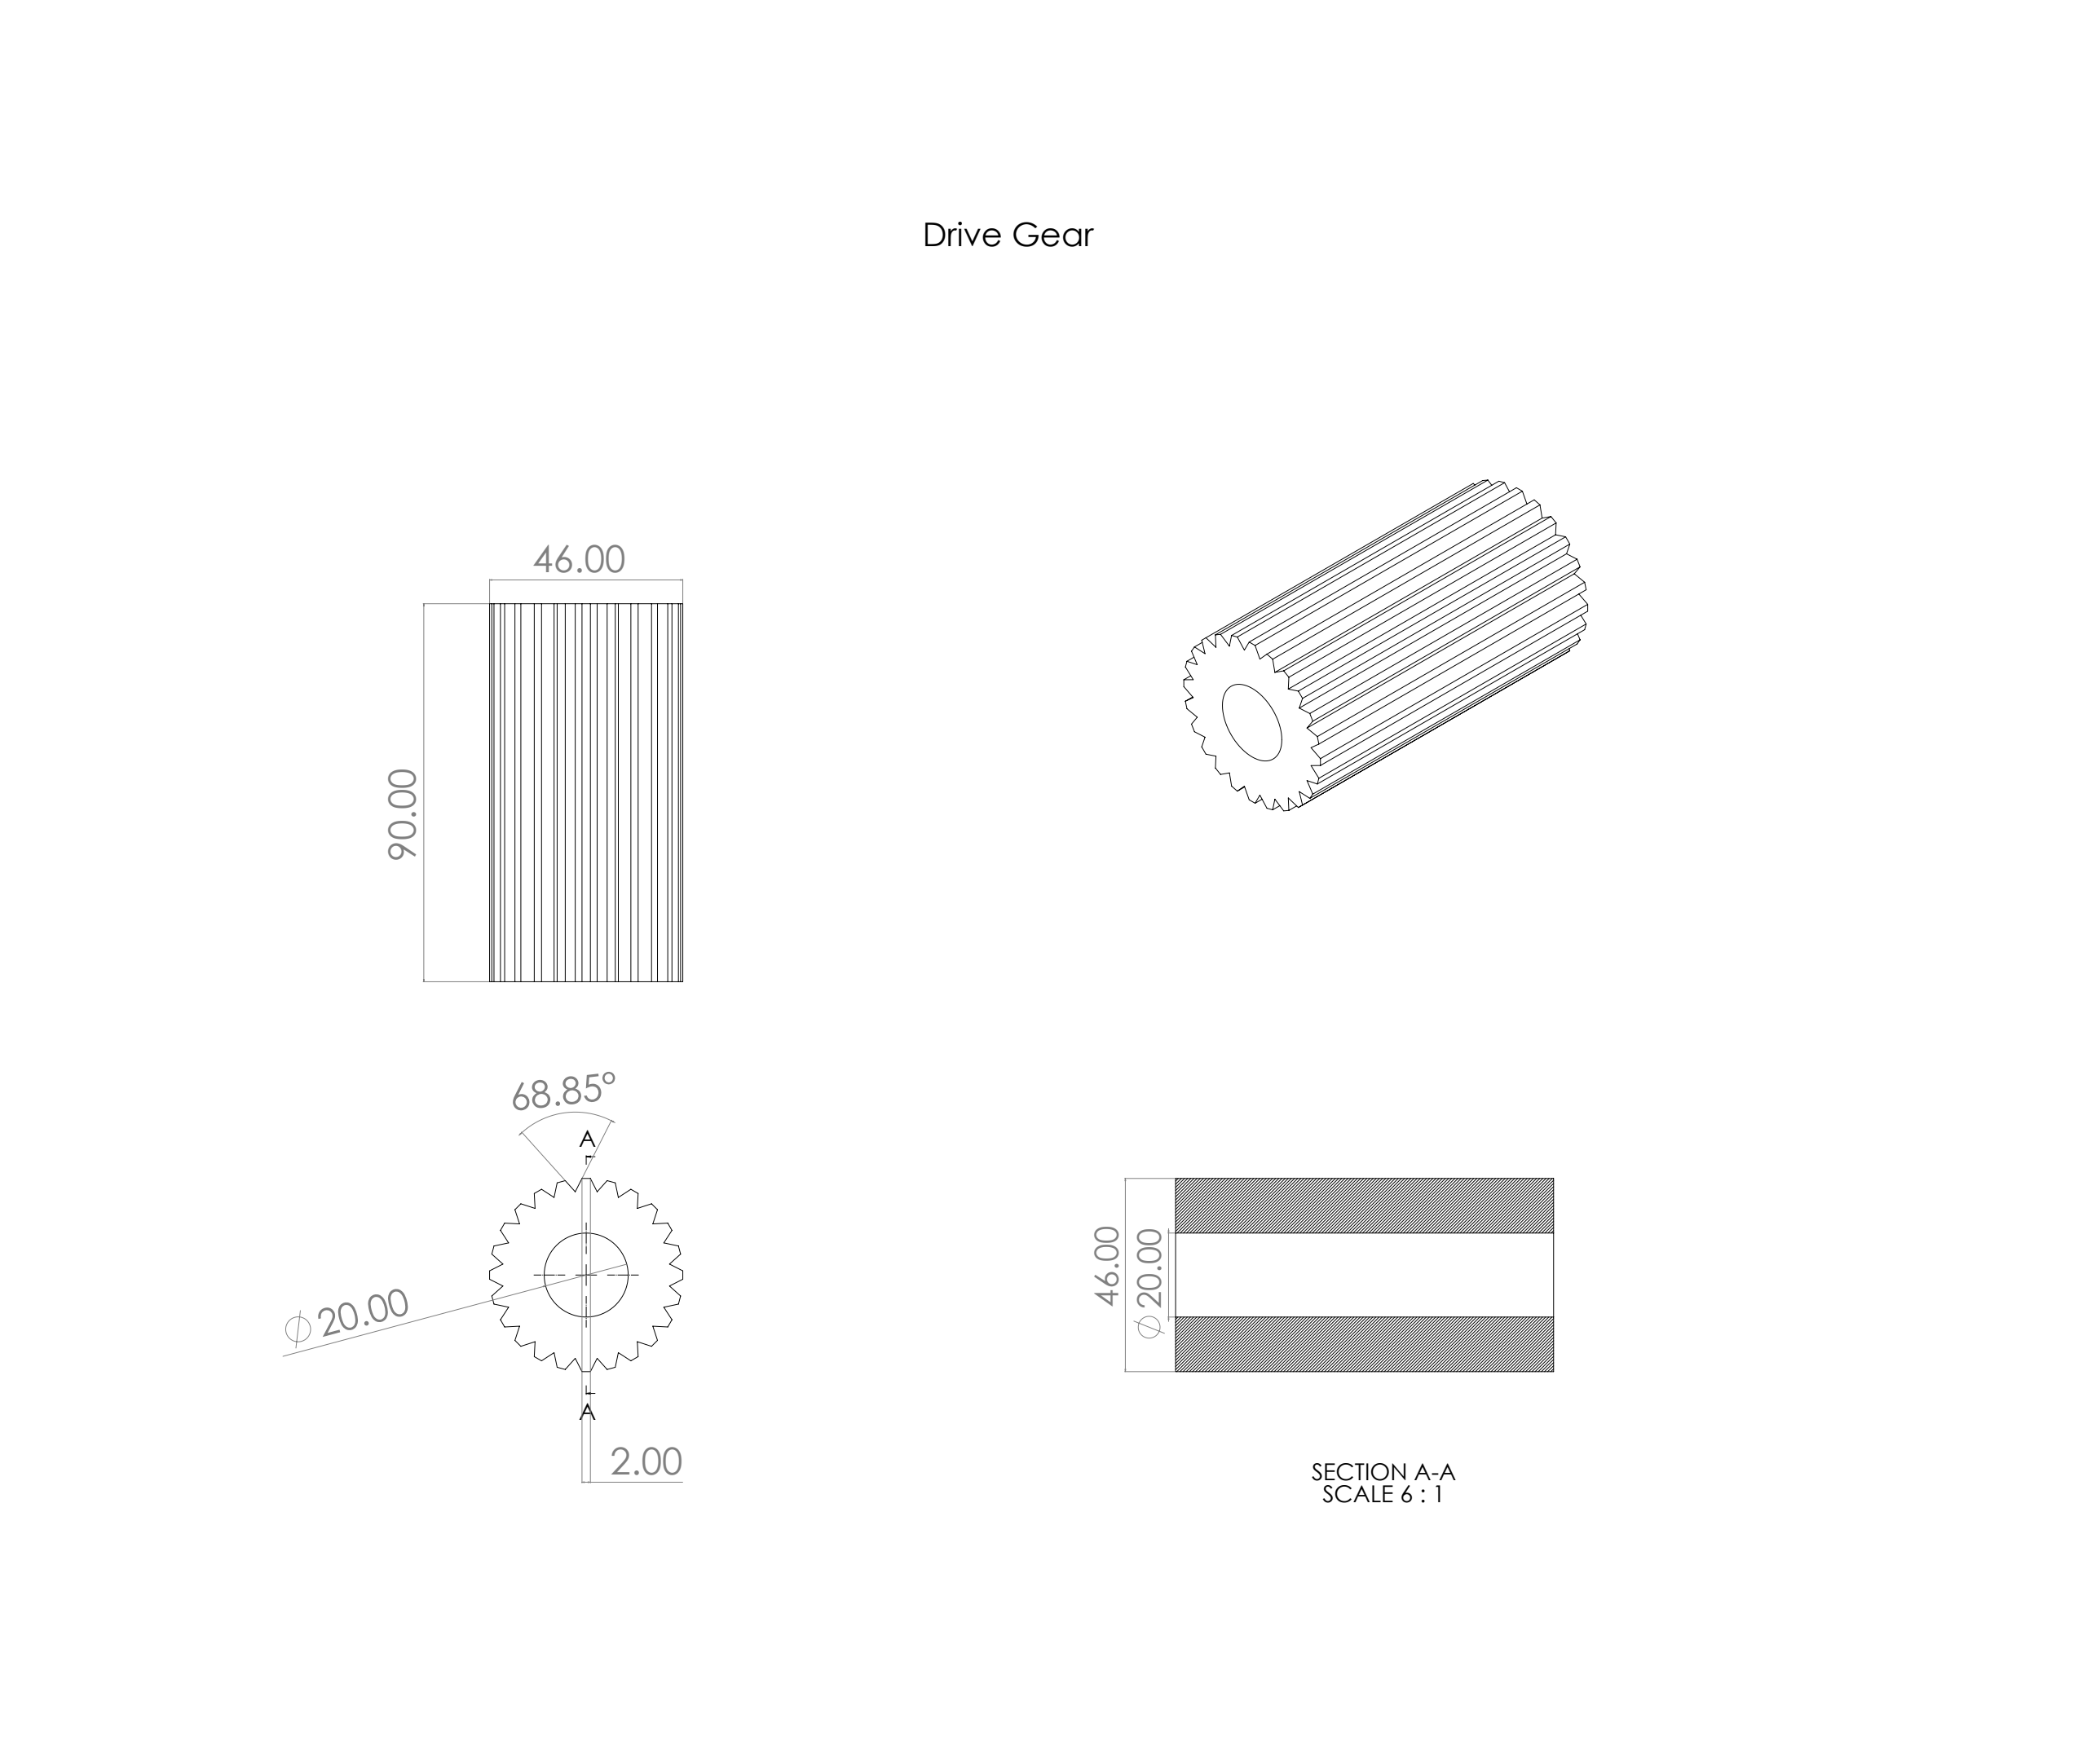
ISO-10303-21;
HEADER;
FILE_DESCRIPTION (('STEP AP214'),
    '1' );
FILE_NAME ('Drive Gear.step',
    '2026-10-24T00:09:50',
    ( '' ),
    ( '' ),
    'SwSTEP 2.0',
    'SolidWorks 2025',
    '' );
FILE_SCHEMA (( 'AUTOMOTIVE_DESIGN' ));
ENDSEC;

DATA;
#40=EDGE_LOOP ( 'NONE', ( #25387, #6950, #12411, #9967 ) ) ;
#42=LINE ( 'NONE', #17847, #25312 ) ;
#78=EDGE_CURVE ( 'NONE', #15009, #7688, #2981, .T. ) ;
#102=LINE ( 'NONE', #19501, #15080 ) ;
#109=EDGE_CURVE ( 'NONE', #28186, #27342, #11484, .T. ) ;
#120=ORIENTED_EDGE ( 'NONE', *, *, #25163, .F. ) ;
#125=PLANE ( 'NONE',  #22915 ) ;
#145=ORIENTED_EDGE ( 'NONE', *, *, #16814, .F. ) ;
#194=VERTEX_POINT ( 'NONE', #10023 ) ;
#196=VECTOR ( 'NONE', #16989, 1000.000000000000000 ) ;
#202=LINE ( 'NONE', #25668, #4520 ) ;
#257=EDGE_LOOP ( 'NONE', ( #18040, #22551, #6751, #26799 ) ) ;
#263=ORIENTED_EDGE ( 'NONE', *, *, #21022, .F. ) ;
#280=CARTESIAN_POINT ( 'NONE',  ( 176.1454027868280434, 57.48855481560072889, -45.00000000000000000 ) ) ;
#290=CARTESIAN_POINT ( 'NONE',  ( 111.3836151241014960, 219.3130464734738325, 45.00000000000000000 ) ) ;
#315=ADVANCED_FACE ( 'NONE', ( #3468 ), #14543, .F. ) ;
#324=CARTESIAN_POINT ( 'NONE',  ( 134.6436608991879496, 206.7391133850113079, 45.00000000000000000 ) ) ;
#338=EDGE_CURVE ( 'NONE', #14636, #5476, #7520, .T. ) ;
#340=EDGE_LOOP ( 'NONE', ( #7547, #3673, #5689, #22912 ) ) ;
#341=ORIENTED_EDGE ( 'NONE', *, *, #16850, .F. ) ;
#343=ADVANCED_FACE ( 'NONE', ( #765 ), #3046, .F. ) ;
#356=AXIS2_PLACEMENT_3D ( 'NONE', #3713, #19096, #27838 ) ;
#395=AXIS2_PLACEMENT_3D ( 'NONE', #17054, #6519, #15304 ) ;
#404=ORIENTED_EDGE ( 'NONE', *, *, #19852, .F. ) ;
#414=VECTOR ( 'NONE', #24913, 999.9999999999998863 ) ;
#421=PLANE ( 'NONE',  #16345 ) ;
#426=CARTESIAN_POINT ( 'NONE',  ( 119.4436508138959567, 203.0294372515225518, 45.00000000000000000 ) ) ;
#460=ORIENTED_EDGE ( 'NONE', *, *, #16342, .F. ) ;
#468=CARTESIAN_POINT ( 'NONE',  ( 157.6866818850739662, 8.471341669691319964, -45.00000000000000000 ) ) ;
#475=DIRECTION ( 'NONE',  ( 0.2066290158914539099, -0.9784193629480814058, 0.000000000000000000 ) ) ;
#481=ORIENTED_EDGE ( 'NONE', *, *, #25209, .F. ) ;
#502=VERTEX_POINT ( 'NONE', #8357 ) ;
#509=ORIENTED_EDGE ( 'NONE', *, *, #9465, .F. ) ;
#551=ORIENTED_EDGE ( 'NONE', *, *, #12670, .T. ) ;
#557=DIRECTION ( 'NONE',  ( -0.9659258262890705327, -0.2588190451025121908, 0.000000000000000000 ) ) ;
#561=CARTESIAN_POINT ( 'NONE',  ( 155.4185842870419947, 230.6339745962152392, -45.00000000000000000 ) ) ;
#570=EDGE_CURVE ( 'NONE', #7917, #3329, #15402, .T. ) ;
#592=AXIS2_PLACEMENT_3D ( 'NONE', #13930, #17784, #13641 ) ;
#599=LINE ( 'NONE', #25008, #4734 ) ;
#609=DIRECTION ( 'NONE',  ( -0.8379557447115514313, 0.5457381880580733924, 0.000000000000000000 ) ) ;
#612=ORIENTED_EDGE ( 'NONE', *, *, #27121, .T. ) ;
#617=LINE ( 'NONE', #13264, #2052 ) ;
#626=CARTESIAN_POINT ( 'NONE',  ( 0.000000000000000000, 0.000000000000000000, 45.00000000000000000 ) ) ;
#627=VERTEX_POINT ( 'NONE', #26725 ) ;
#641=ORIENTED_EDGE ( 'NONE', *, *, #2045, .T. ) ;
#642=LINE ( 'NONE', #11850, #26984 ) ;
#649=LINE ( 'NONE', #27065, #16667 ) ;
#686=CARTESIAN_POINT ( 'NONE',  ( 122.8247714198253959, 235.8670668058242939, 45.00000000000000000 ) ) ;
#694=ORIENTED_EDGE ( 'NONE', *, *, #13779, .T. ) ;
#706=CARTESIAN_POINT ( 'NONE',  ( -56.65306767071049165, 63.08575069354419185, 45.00000000000000000 ) ) ;
#716=AXIS2_PLACEMENT_3D ( 'NONE', #20523, #18375, #3692 ) ;
#718=DIRECTION ( 'NONE',  ( 0.9985600561963489108, -0.05364526231778980747, 0.000000000000000000 ) ) ;
#720=PLANE ( 'NONE',  #20781 ) ;
#732=VECTOR ( 'NONE', #22180, 1000.000000000000000 ) ;
#740=CARTESIAN_POINT ( 'NONE',  ( 145.6339745962154097, 240.4185842870418242, 45.00000000000000000 ) ) ;
#765=FACE_OUTER_BOUND ( 'NONE', #3853, .T. ) ;
#781=DIRECTION ( 'NONE',  ( 0.7071067811865474617, 0.7071067811865474617, 0.000000000000000000 ) ) ;
#788=PLANE ( 'NONE',  #25217 ) ;
#803=ORIENTED_EDGE ( 'NONE', *, *, #16888, .F. ) ;
#809=LINE ( 'NONE', #11602, #22008 ) ;
#810=VECTOR ( 'NONE', #4848, 1000.000000000000000 ) ;
#825=VECTOR ( 'NONE', #26696, 1000.000000000000000 ) ;
#860=VERTEX_POINT ( 'NONE', #14376 ) ;
#884=CARTESIAN_POINT ( 'NONE',  ( -26.22291647523108438, 23.54903675176048594, -45.00000000000000000 ) ) ;
#894=EDGE_CURVE ( 'NONE', #10441, #6349, #7345, .T. ) ;
#900=EDGE_CURVE ( 'NONE', #19228, #8289, #8468, .T. ) ;
#916=VECTOR ( 'NONE', #2379, 1000.000000000000114 ) ;
#950=FACE_OUTER_BOUND ( 'NONE', #5628, .T. ) ;
#951=FACE_OUTER_BOUND ( 'NONE', #17284, .T. ) ;
#953=LINE ( 'NONE', #18483, #6794 ) ;
#962=VERTEX_POINT ( 'NONE', #1425 ) ;
#963=VECTOR ( 'NONE', #22515, 1000.000000000000000 ) ;
#994=CARTESIAN_POINT ( 'NONE',  ( -55.40193461144291831, 169.7519813918499665, 45.00000000000000000 ) ) ;
#999=VERTEX_POINT ( 'NONE', #1707 ) ;
#1002=DIRECTION ( 'NONE',  ( -0.000000000000000000, -0.000000000000000000, -1.000000000000000000 ) ) ;
#1028=ORIENTED_EDGE ( 'NONE', *, *, #14203, .T. ) ;
#1040=ORIENTED_EDGE ( 'NONE', *, *, #11015, .F. ) ;
#1048=CARTESIAN_POINT ( 'NONE',  ( 116.5224093497741364, 227.6536686473013447, 45.00000000000000000 ) ) ;
#1079=EDGE_LOOP ( 'NONE', ( #25472, #803, #15589, #7233 ) ) ;
#1083=ADVANCED_FACE ( 'NONE', ( #13352 ), #125, .F. ) ;
#1084=CARTESIAN_POINT ( 'NONE',  ( 111.9999999999999289, 218.9999999999996874, 45.00000000000000000 ) ) ;
#1090=DIRECTION ( 'NONE',  ( -0.9784193629480828491, -0.2066290158914464437, 0.000000000000000000 ) ) ;
#1092=CARTESIAN_POINT ( 'NONE',  ( -56.65306767071049165, 63.08575069354419185, -45.00000000000000000 ) ) ;
#1094=VECTOR ( 'NONE', #24258, 1000.000000000000000 ) ;
#1102=ORIENTED_EDGE ( 'NONE', *, *, #26834, .F. ) ;
#1115=CARTESIAN_POINT ( 'NONE',  ( -15.28840184913744515, 9.956927649352207865, -45.00000000000000000 ) ) ;
#1118=VECTOR ( 'NONE', #26590, 1000.000000000000114 ) ;
#1121=DIRECTION ( 'NONE',  ( 0.8379557447115634217, 0.5457381880580551847, -0.000000000000000000 ) ) ;
#1126=DIRECTION ( 'NONE',  ( -0.9659258262890652036, 0.2588190451025321748, 0.000000000000000000 ) ) ;
#1135=LINE ( 'NONE', #994, #11133 ) ;
#1148=VECTOR ( 'NONE', #9574, 1000.000000000000000 ) ;
#1152=LINE ( 'NONE', #23410, #5980 ) ;
#1163=DIRECTION ( 'NONE',  ( 0.05364526231778980747, 0.9985600561963489108, -0.000000000000000000 ) ) ;
#1183=DIRECTION ( 'NONE',  ( 0.9506505318133497973, -0.3102637045530707294, 0.000000000000000000 ) ) ;
#1209=ORIENTED_EDGE ( 'NONE', *, *, #3052, .T. ) ;
#1216=EDGE_CURVE ( 'NONE', #7652, #26924, #15939, .T. ) ;
#1218=ORIENTED_EDGE ( 'NONE', *, *, #16788, .T. ) ;
#1234=VECTOR ( 'NONE', #20751, 1000.000000000000000 ) ;
#1238=CARTESIAN_POINT ( 'NONE',  ( 133.9999999999998295, 242.9999999999997158, 45.00000000000000000 ) ) ;
#1259=CARTESIAN_POINT ( 'NONE',  ( 81.39309752945497678, 249.3891174404998594, -45.00000000000000000 ) ) ;
#1260=FACE_OUTER_BOUND ( 'NONE', #1079, .T. ) ;
#1267=ORIENTED_EDGE ( 'NONE', *, *, #22908, .T. ) ;
#1274=CIRCLE ( 'NONE', #5845, 10.00000000000000888 ) ;
#1279=EDGE_LOOP ( 'NONE', ( #24711, #16218, #9881, #10613 ) ) ;
#1302=LINE ( 'NONE', #3588, #3177 ) ;
#1318=DIRECTION ( 'NONE',  ( -0.4999999999999865108, 0.8660254037844464792, 0.000000000000000000 ) ) ;
#1339=EDGE_CURVE ( 'NONE', #6712, #11692, #8855, .T. ) ;
#1341=ADVANCED_FACE ( 'NONE', ( #10873 ), #11018, .F. ) ;
#1345=CARTESIAN_POINT ( 'NONE',  ( 130.0130877889311591, 197.5248869502486571, 45.00000000000000000 ) ) ;
#1355=ORIENTED_EDGE ( 'NONE', *, *, #570, .F. ) ;
#1361=EDGE_LOOP ( 'NONE', ( #16416, #481, #3606, #1446 ) ) ;
#1388=CARTESIAN_POINT ( 'NONE',  ( -54.22951502486254327, 83.26691194124390449, -45.00000000000000000 ) ) ;
#1389=ORIENTED_EDGE ( 'NONE', *, *, #3470, .F. ) ;
#1416=EDGE_LOOP ( 'NONE', ( #15996, #14532, #28328, #12988 ) ) ;
#1418=EDGE_LOOP ( 'NONE', ( #12140, #21492, #17241, #7648 ) ) ;
#1421=ORIENTED_EDGE ( 'NONE', *, *, #8652, .T. ) ;
#1425=CARTESIAN_POINT ( 'NONE',  ( 127.3463313526982716, 201.5224093497739943, 45.00000000000000000 ) ) ;
#1426=DIRECTION ( 'NONE',  ( -0.8660254037844454800, -0.4999999999999881206, 0.000000000000000000 ) ) ;
#1427=DIRECTION ( 'NONE',  ( -0.000000000000000000, -0.000000000000000000, -1.000000000000000000 ) ) ;
#1446=ORIENTED_EDGE ( 'NONE', *, *, #16888, .T. ) ;
#1449=LINE ( 'NONE', #22871, #12208 ) ;
#1466=EDGE_CURVE ( 'NONE', #27470, #21163, #18610, .T. ) ;
#1478=VECTOR ( 'NONE', #2911, 1000.000000000000114 ) ;
#1485=ORIENTED_EDGE ( 'NONE', *, *, #25059, .F. ) ;
#1487=LINE ( 'NONE', #27761, #26260 ) ;
#1498=ORIENTED_EDGE ( 'NONE', *, *, #13064, .T. ) ;
#1530=ORIENTED_EDGE ( 'NONE', *, *, #23337, .F. ) ;
#1551=DIRECTION ( 'NONE',  ( 0.2066290158914464714, -0.9784193629480829602, 0.000000000000000000 ) ) ;
#1553=DIRECTION ( 'NONE',  ( -0.000000000000000000, -0.000000000000000000, -1.000000000000000000 ) ) ;
#1554=VERTEX_POINT ( 'NONE', #1084 ) ;
#1596=ORIENTED_EDGE ( 'NONE', *, *, #15234, .T. ) ;
#1606=PLANE ( 'NONE',  #14436 ) ;
#1621=CARTESIAN_POINT ( 'NONE',  ( 147.1752285801744904, 204.1329331941753082, -45.00000000000000000 ) ) ;
#1629=DIRECTION ( 'NONE',  ( -0.000000000000000000, -0.000000000000000000, -1.000000000000000000 ) ) ;
#1631=ORIENTED_EDGE ( 'NONE', *, *, #5242, .F. ) ;
#1636=ORIENTED_EDGE ( 'NONE', *, *, #26899, .F. ) ;
#1650=CARTESIAN_POINT ( 'NONE',  ( 177.1897033089359184, 197.3087408678716770, 45.00000000000000000 ) ) ;
#1666=DIRECTION ( 'NONE',  ( -0.9784193629480785193, 0.2066290158914672603, 0.000000000000000000 ) ) ;
#1704=ORIENTED_EDGE ( 'NONE', *, *, #7266, .T. ) ;
#1707=CARTESIAN_POINT ( 'NONE',  ( 144.9999999999998863, 220.0000000000000284, -45.00000000000000000 ) ) ;
#1719=ORIENTED_EDGE ( 'NONE', *, *, #1339, .T. ) ;
#1736=VERTEX_POINT ( 'NONE', #1916 ) ;
#1748=CIRCLE ( 'NONE', #20114, 10.00000000000000888 ) ;
#1754=EDGE_CURVE ( 'NONE', #18948, #27470, #15575, .T. ) ;
#1758=SHAPE_REPRESENTATION_RELATIONSHIP ( 'NONE' , 'NONE' ,  #18912, #11228 ) ;
#1763=VECTOR ( 'NONE', #14890, 1000.000000000000000 ) ;
#1765=EDGE_LOOP ( 'NONE', ( #4521, #6128, #4628, #3710 ) ) ;
#1782=VECTOR ( 'NONE', #5929, 1000.000000000000000 ) ;
#1791=LINE ( 'NONE', #13023, #4249 ) ;
#1844=ADVANCED_FACE ( 'NONE', ( #4356 ), #17291, .F. ) ;
#1868=LINE ( 'NONE', #10646, #5333 ) ;
#1869=ORIENTED_EDGE ( 'NONE', *, *, #5831, .T. ) ;
#1870=ORIENTED_EDGE ( 'NONE', *, *, #3281, .F. ) ;
#1885=AXIS2_PLACEMENT_3D ( 'NONE', #20179, #11860, #26790 ) ;
#1887=VECTOR ( 'NONE', #26855, 1000.000000000000114 ) ;
#1892=DIRECTION ( 'NONE',  ( 0.5457381880580697286, -0.8379557447115539848, 0.000000000000000000 ) ) ;
#1897=DIRECTION ( 'NONE',  ( 1.000000000000000000, 0.000000000000000000, 0.000000000000000000 ) ) ;
#1916=CARTESIAN_POINT ( 'NONE',  ( 119.1329331941753225, 207.8247714198252254, -45.00000000000000000 ) ) ;
#1918=CARTESIAN_POINT ( 'NONE',  ( 67.86343429515802939, -22.14858123305036486, -45.00000000000000000 ) ) ;
#1945=EDGE_LOOP ( 'NONE', ( #6961, #13309, #1870, #11630 ) ) ;
#1974=EDGE_LOOP ( 'NONE', ( #18192, #8711 ) ) ;
#1976=AXIS2_PLACEMENT_3D ( 'NONE', #3956, #4099, #27934 ) ;
#2037=PLANE ( 'NONE',  #3279 ) ;
#2045=EDGE_CURVE ( 'NONE', #27342, #12331, #5777, .T. ) ;
#2052=VECTOR ( 'NONE', #18137, 1000.000000000000114 ) ;
#2068=LINE ( 'NONE', #20020, #17266 ) ;
#2075=ADVANCED_FACE ( 'NONE', ( #9953 ), #7662, .F. ) ;
#2089=ORIENTED_EDGE ( 'NONE', *, *, #3406, .F. ) ;
#2117=APPLICATION_CONTEXT ( 'automotive_design' ) ;
#2121=DIRECTION ( 'NONE',  ( -0.9659258262890705327, -0.2588190451025121908, 0.000000000000000000 ) ) ;
#2154=EDGE_CURVE ( 'NONE', #11738, #18634, #27740, .T. ) ;
#2166=ADVANCED_FACE ( 'NONE', ( #14689 ), #9817, .F. ) ;
#2189=ORIENTED_EDGE ( 'NONE', *, *, #1216, .T. ) ;
#2192=VECTOR ( 'NONE', #13945, 1000.000000000000114 ) ;
#2198=DIRECTION ( 'NONE',  ( 1.000000000000000000, 0.000000000000000000, 0.000000000000000000 ) ) ;
#2203=DIRECTION ( 'NONE',  ( 0.9985600561963492439, 0.05364526231778202897, 0.000000000000000000 ) ) ;
#2230=VECTOR ( 'NONE', #25058, 1000.000000000000000 ) ;
#2232=ADVANCED_FACE ( 'NONE', ( #15658 ), #421, .F. ) ;
#2234=EDGE_CURVE ( 'NONE', #24120, #14926, #7170, .T. ) ;
#2235=CARTESIAN_POINT ( 'NONE',  ( 111.3836151241014960, 219.3130464734738325, -45.00000000000000000 ) ) ;
#2237=PLANE ( 'NONE',  #21348 ) ;
#2246=ORIENTED_EDGE ( 'NONE', *, *, #12352, .F. ) ;
#2288=ORIENTED_EDGE ( 'NONE', *, *, #3470, .T. ) ;
#2320=DIRECTION ( 'NONE',  ( 0.000000000000000000, 0.000000000000000000, 1.000000000000000000 ) ) ;
#2324=CARTESIAN_POINT ( 'NONE',  ( 69.99612328191057031, 261.2290884209365345, -45.00000000000000000 ) ) ;
#2379=DIRECTION ( 'NONE',  ( 0.8916010070293484135, -0.4528218681382910060, 0.000000000000000000 ) ) ;
#2401=EDGE_CURVE ( 'NONE', #25350, #8917, #22540, .T. ) ;
#2412=DIRECTION ( 'NONE',  ( 0.6681556583950086781, -0.7440215159219069063, 0.000000000000000000 ) ) ;
#2417=VECTOR ( 'NONE', #27846, 1000.000000000000000 ) ;
#2447=DIRECTION ( 'NONE',  ( -0.9985600561963481336, 0.05364526231780537141, 0.000000000000000000 ) ) ;
#2471=CARTESIAN_POINT ( 'NONE',  ( 8.415662294793918363, -4.274104551145060604, 45.00000000000000000 ) ) ;
#2476=VECTOR ( 'NONE', #18133, 1000.000000000000000 ) ;
#2490=ORIENTED_EDGE ( 'NONE', *, *, #5540, .T. ) ;
#2507=ADVANCED_FACE ( 'NONE', ( #21795 ), #2237, .F. ) ;
#2519=LINE ( 'NONE', #2235, #916 ) ;
#2554=UNCERTAINTY_MEASURE_WITH_UNIT (LENGTH_MEASURE( 1.000000000000000082E-05 ), #11582, 'distance_accuracy_value', 'NONE');
#2558=DIRECTION ( 'NONE',  ( 0.3102637045530588500, -0.9506505318133536830, 0.000000000000000000 ) ) ;
#2564=LINE ( 'NONE', #426, #825 ) ;
#2570=DIRECTION ( 'NONE',  ( -0.000000000000000000, -0.000000000000000000, -1.000000000000000000 ) ) ;
#2571=DIRECTION ( 'NONE',  ( -0.8660254037844394848, 0.4999999999999985012, 0.000000000000000000 ) ) ;
#2580=AXIS2_PLACEMENT_3D ( 'NONE', #15107, #13103, #3886 ) ;
#2587=ORIENTED_EDGE ( 'NONE', *, *, #26111, .F. ) ;
#2592=CARTESIAN_POINT ( 'NONE',  ( 161.2365440327092472, 161.2365440327092472, 45.00000000000000000 ) ) ;
#2611=VERTEX_POINT ( 'NONE', #23070 ) ;
#2612=CARTESIAN_POINT ( 'NONE',  ( 119.4436508138959567, 203.0294372515225518, -45.00000000000000000 ) ) ;
#2654=ORIENTED_EDGE ( 'NONE', *, *, #23931, .T. ) ;
#2666=DIRECTION ( 'NONE',  ( 0.2066290158914672881, 0.9784193629480785193, 0.000000000000000000 ) ) ;
#2679=EDGE_CURVE ( 'NONE', #24350, #28016, #12165, .T. ) ;
#2681=LINE ( 'NONE', #5123, #20173 ) ;
#2710=CARTESIAN_POINT ( 'NONE',  ( 122.8247714198256944, 204.1329331941749672, 45.00000000000000000 ) ) ;
#2712=VECTOR ( 'NONE', #22898, 999.9999999999998863 ) ;
#2721=VECTOR ( 'NONE', #7878, 1000.000000000000000 ) ;
#2725=VECTOR ( 'NONE', #21249, 999.9999999999998863 ) ;
#2732=ADVANCED_FACE ( 'NONE', ( #20765 ), #9855, .F. ) ;
#2745=LINE ( 'NONE', #18132, #9284 ) ;
#2746=LINE ( 'NONE', #7067, #18086 ) ;
#2762=DIRECTION ( 'NONE',  ( 0.9985600561963485777, -0.05364526231779676024, 0.000000000000000000 ) ) ;
#2779=CARTESIAN_POINT ( 'NONE',  ( 132.3894761555990556, 200.1711027725235397, 45.00000000000000000 ) ) ;
#2780=DIRECTION ( 'NONE',  ( -0.7071067811865614505, -0.7071067811865336949, 0.000000000000000000 ) ) ;
#2792=ORIENTED_EDGE ( 'NONE', *, *, #22790, .F. ) ;
#2801=CARTESIAN_POINT ( 'NONE',  ( 157.9999999999998579, 219.0000000000000284, -45.00000000000000000 ) ) ;
#2814=DIRECTION ( 'NONE',  ( -0.9659258262890670910, 0.2588190451025251804, 0.000000000000000000 ) ) ;
#2817=PLANE ( 'NONE',  #28111 ) ;
#2823=LINE ( 'NONE', #11617, #23613 ) ;
#2845=LINE ( 'NONE', #20656, #9838 ) ;
#2847=LINE ( 'NONE', #11639, #4974 ) ;
#2850=CARTESIAN_POINT ( 'NONE',  ( 151.9705627484769650, 235.5563491861038017, 45.00000000000000000 ) ) ;
#2870=ORIENTED_EDGE ( 'NONE', *, *, #14550, .T. ) ;
#2873=VERTEX_POINT ( 'NONE', #10139 ) ;
#2890=EDGE_CURVE ( 'NONE', #24769, #999, #18891, .T. ) ;
#2902=FACE_OUTER_BOUND ( 'NONE', #28230, .T. ) ;
#2910=ORIENTED_EDGE ( 'NONE', *, *, #25628, .T. ) ;
#2911=DIRECTION ( 'NONE',  ( 0.05364526231776645809, -0.9985600561963501320, 0.000000000000000000 ) ) ;
#2925=DIRECTION ( 'NONE',  ( -0.000000000000000000, -0.000000000000000000, -1.000000000000000000 ) ) ;
#2927=CARTESIAN_POINT ( 'NONE',  ( 46.36636626309694975, -15.13258561588589757, -45.00000000000000000 ) ) ;
#2930=DIRECTION ( 'NONE',  ( 0.2588190451024993122, -0.9659258262890740854, 0.000000000000000000 ) ) ;
#2939=VERTEX_POINT ( 'NONE', #15446 ) ;
#2940=DIRECTION ( 'NONE',  ( -0.000000000000000000, -0.000000000000000000, -1.000000000000000000 ) ) ;
#2968=DIRECTION ( 'NONE',  ( -0.000000000000000000, -0.000000000000000000, -1.000000000000000000 ) ) ;
#2976=ORIENTED_EDGE ( 'NONE', *, *, #25059, .T. ) ;
#2981=LINE ( 'NONE', #7160, #15959 ) ;
#2988=DIRECTION ( 'NONE',  ( -0.000000000000000000, -0.000000000000000000, -1.000000000000000000 ) ) ;
#3005=EDGE_CURVE ( 'NONE', #27691, #16717, #15580, .T. ) ;
#3015=VECTOR ( 'NONE', #6084, 1000.000000000000000 ) ;
#3035=ORIENTED_EDGE ( 'NONE', *, *, #2045, .F. ) ;
#3046=PLANE ( 'NONE',  #15104 ) ;
#3052=EDGE_CURVE ( 'NONE', #24120, #16717, #26777, .T. ) ;
#3063=DIRECTION ( 'NONE',  ( -0.4999999999999985012, -0.8660254037844394848, 0.000000000000000000 ) ) ;
#3070=ORIENTED_EDGE ( 'NONE', *, *, #1754, .F. ) ;
#3088=CIRCLE ( 'NONE', #356, 10.00000000000000888 ) ;
#3091=CARTESIAN_POINT ( 'NONE',  ( 193.7634559672933676, 193.7634559672857790, 45.00000000000000000 ) ) ;
#3092=CARTESIAN_POINT ( 'NONE',  ( -26.23654403271235225, 26.23654403271337543, 45.00000000000000000 ) ) ;
#3123=VECTOR ( 'NONE', #22798, 1000.000000000000000 ) ;
#3133=DIRECTION ( 'NONE',  ( 0.000000000000000000, -0.000000000000000000, -1.000000000000000000 ) ) ;
#3138=DIRECTION ( 'NONE',  ( -0.9985600561963485777, -0.05364526231779759985, 0.000000000000000000 ) ) ;
#3157=VECTOR ( 'NONE', #2121, 1000.000000000000114 ) ;
#3177=VECTOR ( 'NONE', #21120, 1000.000000000000114 ) ;
#3182=FACE_OUTER_BOUND ( 'NONE', #20955, .T. ) ;
#3242=LINE ( 'NONE', #18765, #15841 ) ;
#3264=CARTESIAN_POINT ( 'NONE',  ( 185.9255560592262100, 121.0883471088020116, 45.00000000000000000 ) ) ;
#3279=AXIS2_PLACEMENT_3D ( 'NONE', #8516, #21866, #17268 ) ;
#3281=EDGE_CURVE ( 'NONE', #10285, #27697, #26871, .T. ) ;
#3300=EDGE_CURVE ( 'NONE', #7395, #1554, #9777, .T. ) ;
#3309=EDGE_CURVE ( 'NONE', #7097, #3365, #25132, .T. ) ;
#3311=PLANE ( 'NONE',  #21814 ) ;
#3326=DIRECTION ( 'NONE',  ( 1.387778780781444413E-14, 1.000000000000000000, 0.000000000000000000 ) ) ;
#3329=VERTEX_POINT ( 'NONE', #17790 ) ;
#3334=CARTESIAN_POINT ( 'NONE',  ( -43.04748092857122543, 38.65804596583237895, 45.00000000000000000 ) ) ;
#3339=EDGE_CURVE ( 'NONE', #20334, #27997, #18371, .T. ) ;
#3342=DIRECTION ( 'NONE',  ( -0.7440215159219069063, -0.6681556583950086781, 0.000000000000000000 ) ) ;
#3343=LINE ( 'NONE', #10247, #5075 ) ;
#3350=VERTEX_POINT ( 'NONE', #24402 ) ;
#3365=VERTEX_POINT ( 'NONE', #22247 ) ;
#3369=VECTOR ( 'NONE', #15588, 1000.000000000000000 ) ;
#3376=ADVANCED_FACE ( 'NONE', ( #22106 ), #6876, .F. ) ;
#3405=VECTOR ( 'NONE', #9865, 1000.000000000000000 ) ;
#3406=EDGE_CURVE ( 'NONE', #26858, #28003, #5000, .T. ) ;
#3410=CARTESIAN_POINT ( 'NONE',  ( 119.4436508138957720, 236.9705627484767376, 45.00000000000000000 ) ) ;
#3415=FACE_OUTER_BOUND ( 'NONE', #6007, .T. ) ;
#3421=ORIENTED_EDGE ( 'NONE', *, *, #26111, .T. ) ;
#3439=EDGE_CURVE ( 'NONE', #1554, #13479, #2847, .T. ) ;
#3460=EDGE_CURVE ( 'NONE', #16717, #18830, #27813, .T. ) ;
#3468=FACE_OUTER_BOUND ( 'NONE', #28210, .T. ) ;
#3470=EDGE_CURVE ( 'NONE', #21880, #27997, #25394, .T. ) ;
#3472=ORIENTED_EDGE ( 'NONE', *, *, #26710, .T. ) ;
#3475=EDGE_CURVE ( 'NONE', #3728, #10441, #23379, .T. ) ;
#3496=VERTEX_POINT ( 'NONE', #9889 ) ;
#3512=ADVANCED_FACE ( 'NONE', ( #1260 ), #16502, .F. ) ;
#3523=EDGE_LOOP ( 'NONE', ( #17931, #11794, #13410, #15572 ) ) ;
#3524=DIRECTION ( 'NONE',  ( 0.9985600561963481336, -0.05364526231780537141, 0.000000000000000000 ) ) ;
#3531=PLANE ( 'NONE',  #11762 ) ;
#3554=CARTESIAN_POINT ( 'NONE',  ( -26.23654403271235225, 26.23654403271337543, -45.00000000000000000 ) ) ;
#3561=VECTOR ( 'NONE', #21819, 1000.000000000000000 ) ;
#3579=DIRECTION ( 'NONE',  ( -0.000000000000000000, -0.000000000000000000, -1.000000000000000000 ) ) ;
#3585=CARTESIAN_POINT ( 'NONE',  ( 150.8670668058245212, 232.1752285801742630, 45.00000000000000000 ) ) ;
#3588=CARTESIAN_POINT ( 'NONE',  ( -43.04748092857122543, 38.65804596583237895, -45.00000000000000000 ) ) ;
#3606=ORIENTED_EDGE ( 'NONE', *, *, #18957, .F. ) ;
#3613=CARTESIAN_POINT ( 'NONE',  ( 115.1711027725237955, 217.3894761555985156, -45.00000000000000000 ) ) ;
#3639=EDGE_CURVE ( 'NONE', #22969, #27280, #17578, .T. ) ;
#3640=VECTOR ( 'NONE', #17767, 1000.000000000000114 ) ;
#3649=VERTEX_POINT ( 'NONE', #13151 ) ;
#3666=EDGE_CURVE ( 'NONE', #15219, #4484, #202, .T. ) ;
#3673=ORIENTED_EDGE ( 'NONE', *, *, #23039, .F. ) ;
#3674=EDGE_CURVE ( 'NONE', #24234, #24769, #1748, .T. ) ;
#3677=ORIENTED_EDGE ( 'NONE', *, *, #15337, .F. ) ;
#3682=ORIENTED_EDGE ( 'NONE', *, *, #11254, .T. ) ;
#3687=DIRECTION ( 'NONE',  ( -0.000000000000000000, -0.000000000000000000, -1.000000000000000000 ) ) ;
#3692=DIRECTION ( 'NONE',  ( 0.8916010070293515222, -0.4528218681382848443, 0.000000000000000000 ) ) ;
#3710=ORIENTED_EDGE ( 'NONE', *, *, #8134, .T. ) ;
#3713=CARTESIAN_POINT ( 'NONE',  ( 134.9999999999998579, 220.0000000000000284, 45.00000000000000000 ) ) ;
#3717=EDGE_CURVE ( 'NONE', #6540, #10285, #26468, .T. ) ;
#3728=VERTEX_POINT ( 'NONE', #22322 ) ;
#3744=AXIS2_PLACEMENT_3D ( 'NONE', #15881, #2780, #28028 ) ;
#3756=FACE_OUTER_BOUND ( 'NONE', #11512, .T. ) ;
#3759=ADVANCED_FACE ( 'NONE', ( #10449 ), #19207, .F. ) ;
#3786=ORIENTED_EDGE ( 'NONE', *, *, #2679, .F. ) ;
#3811=CARTESIAN_POINT ( 'NONE',  ( 0.000000000000000000, 196.9999999999997442, 45.00000000000000000 ) ) ;
#3843=PLANE ( 'NONE',  #16875 ) ;
#3848=CARTESIAN_POINT ( 'NONE',  ( 157.4751130497510303, 215.0130877889310455, -45.00000000000000000 ) ) ;
#3850=ORIENTED_EDGE ( 'NONE', *, *, #17554, .T. ) ;
#3853=EDGE_LOOP ( 'NONE', ( #11519, #4209, #23044, #8212 ) ) ;
#3880=VERTEX_POINT ( 'NONE', #13717 ) ;
#3885=CARTESIAN_POINT ( 'NONE',  ( 113.0425250404539241, 213.0812361363525440, -45.00000000000000000 ) ) ;
#3886=DIRECTION ( 'NONE',  ( 0.000000000000000000, 0.000000000000000000, 1.000000000000000000 ) ) ;
#3899=CARTESIAN_POINT ( 'NONE',  ( 12.78000883847031588, 237.8887863075477469, 45.00000000000000000 ) ) ;
#3915=DIRECTION ( 'NONE',  ( -0.000000000000000000, -0.000000000000000000, -1.000000000000000000 ) ) ;
#3917=ORIENTED_EDGE ( 'NONE', *, *, #27423, .F. ) ;
#3928=DIRECTION ( 'NONE',  ( -0.8660254037844326014, 0.5000000000000106581, 0.000000000000000000 ) ) ;
#3947=ORIENTED_EDGE ( 'NONE', *, *, #18957, .T. ) ;
#3949=FACE_OUTER_BOUND ( 'NONE', #13104, .T. ) ;
#3953=CARTESIAN_POINT ( 'NONE',  ( 58.09044720719344213, 216.7965004116395562, -45.00000000000000000 ) ) ;
#3956=CARTESIAN_POINT ( 'NONE',  ( -50.01279441628821587, 86.62470095750859400, 45.00000000000000000 ) ) ;
#3965=ORIENTED_EDGE ( 'NONE', *, *, #5540, .F. ) ;
#3990=ORIENTED_EDGE ( 'NONE', *, *, #6896, .T. ) ;
#4010=CARTESIAN_POINT ( 'NONE',  ( 139.9869122110687840, 242.4751130497508314, 45.00000000000000000 ) ) ;
#4021=ORIENTED_EDGE ( 'NONE', *, *, #21820, .T. ) ;
#4035=EDGE_LOOP ( 'NONE', ( #12323, #19079, #7438, #21841 ) ) ;
#4052=DIRECTION ( 'NONE',  ( 0.9506505318133482429, -0.3102637045530752258, 0.000000000000000000 ) ) ;
#4065=VECTOR ( 'NONE', #21116, 1000.000000000000114 ) ;
#4095=CARTESIAN_POINT ( 'NONE',  ( 150.5563491861038870, 236.9705627484768797, 45.00000000000000000 ) ) ;
#4099=DIRECTION ( 'NONE',  ( -0.4999999999999985012, 0.8660254037844394848, 0.000000000000000000 ) ) ;
#4104=CARTESIAN_POINT ( 'NONE',  ( 145.6339745962156940, 199.5814157129578064, -45.00000000000000000 ) ) ;
#4131=VECTOR ( 'NONE', #18316, 999.9999999999998863 ) ;
#4132=APPLICATION_CONTEXT ( 'automotive_design' ) ;
#4146=CARTESIAN_POINT ( 'NONE',  ( 147.3660254037845334, 200.5814157129577779, 45.00000000000000000 ) ) ;
#4172=LINE ( 'NONE', #24394, #23531 ) ;
#4179=VECTOR ( 'NONE', #1090, 1000.000000000000114 ) ;
#4197=ORIENTED_EDGE ( 'NONE', *, *, #10242, .T. ) ;
#4208=FACE_OUTER_BOUND ( 'NONE', #12784, .T. ) ;
#4209=ORIENTED_EDGE ( 'NONE', *, *, #17885, .F. ) ;
#4231=ORIENTED_EDGE ( 'NONE', *, *, #7155, .F. ) ;
#4239=DIRECTION ( 'NONE',  ( -0.000000000000000000, -0.000000000000000000, -1.000000000000000000 ) ) ;
#4249=VECTOR ( 'NONE', #28071, 1000.000000000000114 ) ;
#4268=ORIENTED_EDGE ( 'NONE', *, *, #17273, .F. ) ;
#4269=AXIS2_PLACEMENT_3D ( 'NONE', #18991, #12687, #5774 ) ;
#4274=CARTESIAN_POINT ( 'NONE',  ( 186.0596930950812293, 94.49506802741289846, 45.00000000000000000 ) ) ;
#4289=DIRECTION ( 'NONE',  ( 1.000000000000000000, 0.000000000000000000, 0.000000000000000000 ) ) ;
#4303=FACE_OUTER_BOUND ( 'NONE', #21706, .T. ) ;
#4313=ORIENTED_EDGE ( 'NONE', *, *, #23337, .T. ) ;
#4343=LINE ( 'NONE', #6359, #17050 ) ;
#4356=FACE_OUTER_BOUND ( 'NONE', #18639, .T. ) ;
#4357=VECTOR ( 'NONE', #15478, 999.9999999999998863 ) ;
#4386=ORIENTED_EDGE ( 'NONE', *, *, #9623, .F. ) ;
#4424=CARTESIAN_POINT ( 'NONE',  ( 124.3660254037843771, 240.4185842870417105, -45.00000000000000000 ) ) ;
#4475=ADVANCED_FACE ( 'NONE', ( #13361 ), #24265, .F. ) ;
#4477=DIRECTION ( 'NONE',  ( -0.5457381880580697286, 0.8379557447115539848, 0.000000000000000000 ) ) ;
#4484=VERTEX_POINT ( 'NONE', #21686 ) ;
#4511=CARTESIAN_POINT ( 'NONE',  ( -50.01279441628821587, 86.62470095750859400, 45.00000000000000000 ) ) ;
#4520=VECTOR ( 'NONE', #5991, 1000.000000000000000 ) ;
#4521=ORIENTED_EDGE ( 'NONE', *, *, #14366, .T. ) ;
#4525=VERTEX_POINT ( 'NONE', #15086 ) ;
#4542=FACE_OUTER_BOUND ( 'NONE', #17105, .T. ) ;
#4554=VERTEX_POINT ( 'NONE', #20238 ) ;
#4561=ORIENTED_EDGE ( 'NONE', *, *, #16547, .F. ) ;
#4575=CARTESIAN_POINT ( 'NONE',  ( 135.1062353973271968, 7.258260926501912458, 45.00000000000000000 ) ) ;
#4583=VERTEX_POINT ( 'NONE', #2710 ) ;
#4628=ORIENTED_EDGE ( 'NONE', *, *, #21147, .F. ) ;
#4630=PLANE ( 'NONE',  #13448 ) ;
#4631=EDGE_CURVE ( 'NONE', #27697, #7917, #24407, .T. ) ;
#4632=VECTOR ( 'NONE', #2570, 1000.000000000000000 ) ;
#4652=ORIENTED_EDGE ( 'NONE', *, *, #15149, .T. ) ;
#4655=EDGE_CURVE ( 'NONE', #21098, #10156, #2564, .T. ) ;
#4656=VECTOR ( 'NONE', #1629, 1000.000000000000000 ) ;
#4669=ADVANCED_FACE ( 'NONE', ( #3415 ), #3843, .F. ) ;
#4686=ADVANCED_FACE ( 'NONE', ( #12486 ), #10178, .F. ) ;
#4697=VECTOR ( 'NONE', #1553, 1000.000000000000000 ) ;
#4701=ORIENTED_EDGE ( 'NONE', *, *, #20546, .F. ) ;
#4705=LINE ( 'NONE', #24830, #810 ) ;
#4725=CARTESIAN_POINT ( 'NONE',  ( 154.8288972274760908, 217.3894761555990556, 45.00000000000000000 ) ) ;
#4734=VECTOR ( 'NONE', #27013, 999.9999999999998863 ) ;
#4759=LINE ( 'NONE', #8163, #18997 ) ;
#4773=DIRECTION ( 'NONE',  ( 0.05364526231779676024, 0.9985600561963485777, 0.000000000000000000 ) ) ;
#4776=VERTEX_POINT ( 'NONE', #18792 ) ;
#4777=VECTOR ( 'NONE', #16926, 999.9999999999998863 ) ;
#4798=PLANE ( 'NONE',  #12083 ) ;
#4811=CARTESIAN_POINT ( 'NONE',  ( 111.9999999999968878, -1.554312234475174324E-12, -45.00000000000000000 ) ) ;
#4816=AXIS2_PLACEMENT_3D ( 'NONE', #12746, #27800, #23506 ) ;
#4830=ORIENTED_EDGE ( 'NONE', *, *, #24113, .T. ) ;
#4831=LINE ( 'NONE', #8727, #15638 ) ;
#4836=VERTEX_POINT ( 'NONE', #10885 ) ;
#4848=DIRECTION ( 'NONE',  ( -0.000000000000000000, -0.000000000000000000, -1.000000000000000000 ) ) ;
#4851=AXIS2_PLACEMENT_3D ( 'NONE', #27456, #23443, #12932 ) ;
#4859=DIRECTION ( 'NONE',  ( 0.5457381880580733924, 0.8379557447115514313, 0.000000000000000000 ) ) ;
#4873=EDGE_CURVE ( 'NONE', #23798, #14035, #102, .T. ) ;
#4880=VECTOR ( 'NONE', #6475, 1000.000000000000114 ) ;
#4882=DIRECTION ( 'NONE',  ( 0.5457381880580733924, 0.8379557447115515423, -0.000000000000000000 ) ) ;
#4886=CARTESIAN_POINT ( 'NONE',  ( 151.9705627484771355, 204.4436508138959141, 45.00000000000000000 ) ) ;
#4889=DIRECTION ( 'NONE',  ( -0.7071067811865474617, 0.7071067811865474617, 0.000000000000000000 ) ) ;
#4903=LINE ( 'NONE', #26893, #12393 ) ;
#4915=FACE_BOUND ( 'NONE', #23866, .T. ) ;
#4922=LINE ( 'NONE', #11267, #5239 ) ;
#4929=DIRECTION ( 'NONE',  ( -0.000000000000000000, -0.000000000000000000, -1.000000000000000000 ) ) ;
#4931=DIRECTION ( 'NONE',  ( -0.9659258262890740854, -0.2588190451024993122, 0.000000000000000000 ) ) ;
#4937=CARTESIAN_POINT ( 'NONE',  ( -51.90955279280624524, 193.7290884209386661, 45.00000000000000000 ) ) ;
#4942=( NAMED_UNIT ( * ) SI_UNIT ( $, .STERADIAN. ) SOLID_ANGLE_UNIT ( ) );
#4956=ORIENTED_EDGE ( 'NONE', *, *, #9850, .F. ) ;
#4963=CARTESIAN_POINT ( 'NONE',  ( 175.6862808370088089, 157.7720269260891826, 45.00000000000000000 ) ) ;
#4974=VECTOR ( 'NONE', #20378, 1000.000000000000114 ) ;
#4982=VERTEX_POINT ( 'NONE', #22221 ) ;
#4986=ORIENTED_EDGE ( 'NONE', *, *, #5214, .T. ) ;
#4991=FACE_OUTER_BOUND ( 'NONE', #4035, .T. ) ;
#5000=LINE ( 'NONE', #280, #26518 ) ;
#5013=LINE ( 'NONE', #4725, #9308 ) ;
#5027=DIRECTION ( 'NONE',  ( -1.387778780781444256E-14, -1.000000000000000000, 0.000000000000000000 ) ) ;
#5058=ORIENTED_EDGE ( 'NONE', *, *, #24113, .F. ) ;
#5075=VECTOR ( 'NONE', #7807, 1000.000000000000114 ) ;
#5085=ORIENTED_EDGE ( 'NONE', *, *, #23141, .T. ) ;
#5090=CARTESIAN_POINT ( 'NONE',  ( 151.9705627484769650, 235.5563491861038017, -45.00000000000000000 ) ) ;
#5103=ORIENTED_EDGE ( 'NONE', *, *, #6236, .T. ) ;
#5109=DIRECTION ( 'NONE',  ( -0.9784193629480781862, 0.2066290158914688424, 0.000000000000000000 ) ) ;
#5111=CARTESIAN_POINT ( 'NONE',  ( 118.0294372515228787, 204.4436508138956015, 45.00000000000000000 ) ) ;
#5123=CARTESIAN_POINT ( 'NONE',  ( 155.4185842870419947, 230.6339745962152392, 45.00000000000000000 ) ) ;
#5124=CARTESIAN_POINT ( 'NONE',  ( 162.0806940948679085, 180.4841764145329250, 45.00000000000000000 ) ) ;
#5159=CARTESIAN_POINT ( 'NONE',  ( 133.9999999999998295, 242.9999999999997158, 45.00000000000000000 ) ) ;
#5160=DIRECTION ( 'NONE',  ( -0.7440215159219069063, -0.6681556583950086781, 0.000000000000000000 ) ) ;
#5166=AXIS2_PLACEMENT_3D ( 'NONE', #25267, #12218, #18803 ) ;
#5169=VERTEX_POINT ( 'NONE', #7573 ) ;
#5183=VECTOR ( 'NONE', #14605, 1000.000000000000000 ) ;
#5190=LINE ( 'NONE', #27431, #2476 ) ;
#5206=CARTESIAN_POINT ( 'NONE',  ( 135.1062353973271968, 7.258260926501912458, 45.00000000000000000 ) ) ;
#5210=ORIENTED_EDGE ( 'NONE', *, *, #13674, .T. ) ;
#5214=EDGE_CURVE ( 'NONE', #19703, #15612, #27645, .T. ) ;
#5239=VECTOR ( 'NONE', #19731, 1000.000000000000000 ) ;
#5240=EDGE_CURVE ( 'NONE', #28016, #27342, #25222, .T. ) ;
#5242=EDGE_CURVE ( 'NONE', #502, #26105, #953, .T. ) ;
#5266=EDGE_CURVE ( 'NONE', #3350, #19969, #16337, .T. ) ;
#5283=EDGE_LOOP ( 'NONE', ( #2288, #13556, #20817, #3682 ) ) ;
#5285=CARTESIAN_POINT ( 'NONE',  ( 150.8670668058247202, 207.8247714198255949, -45.00000000000000000 ) ) ;
#5311=FACE_OUTER_BOUND ( 'NONE', #5646, .T. ) ;
#5331=CARTESIAN_POINT ( 'NONE',  ( 192.5108452903457419, 172.8810361401565672, 45.00000000000000000 ) ) ;
#5333=VECTOR ( 'NONE', #25721, 1000.000000000000114 ) ;
#5336=LINE ( 'NONE', #16544, #26391 ) ;
#5349=CARTESIAN_POINT ( 'NONE',  ( 216.4313787033304379, 124.9567147554451623, 45.00000000000000000 ) ) ;
#5376=VERTEX_POINT ( 'NONE', #19462 ) ;
#5401=DIRECTION ( 'NONE',  ( -0.4528218681382693567, 0.8916010070293595158, 0.000000000000000000 ) ) ;
#5424=DIRECTION ( 'NONE',  ( -0.8660254037844454800, -0.4999999999999881206, 0.000000000000000000 ) ) ;
#5430=VECTOR ( 'NONE', #15578, 1000.000000000000114 ) ;
#5433=CARTESIAN_POINT ( 'NONE',  ( 186.0596930950812293, 94.49506802741289846, 45.00000000000000000 ) ) ;
#5436=PLANE ( 'NONE',  #14659 ) ;
#5439=ORIENTED_EDGE ( 'NONE', *, *, #22847, .T. ) ;
#5444=EDGE_LOOP ( 'NONE', ( #7202, #15181, #8500, #25324, #13483, #17674, #19369, #2587, #23358, #460, #9912, #24920, #263, #8980, #25934, #23719, #3070, #8562, #25601, #1040, #13343, #19688, #22529, #27521, #28362, #4701, #14695, #19614, #21863, #18695, #27803, #22872, #25095, #23438, #24915, #9168, #7561, #12434, #15681, #1485, #1530, #22418, #23738, #1389, #22616, #2089, #16211, #20617, #28380, #23974, #9500, #4386, #17629, #509, #20850, #8253, #5870, #341, #12391, #27763, #10263, #16896, #19293, #3035, #27917, #12006, #23575, #16998, #13544, #3917, #13144, #28340 ) ) ;
#5453=VECTOR ( 'NONE', #24288, 1000.000000000000000 ) ;
#5470=CARTESIAN_POINT ( 'NONE',  ( 116.5224093497741364, 227.6536686473013447, 45.00000000000000000 ) ) ;
#5476=VERTEX_POINT ( 'NONE', #13293 ) ;
#5483=ORIENTED_EDGE ( 'NONE', *, *, #7657, .T. ) ;
#5489=ORIENTED_EDGE ( 'NONE', *, *, #2154, .F. ) ;
#5494=DIRECTION ( 'NONE',  ( -0.8379557447115549840, -0.5457381880580680633, 0.000000000000000000 ) ) ;
#5504=DIRECTION ( 'NONE',  ( -0.6681556583950086781, 0.7440215159219069063, 0.000000000000000000 ) ) ;
#5508=CARTESIAN_POINT ( 'NONE',  ( -66.26041567618258910, 130.4659900502583127, 45.00000000000000000 ) ) ;
#5513=DIRECTION ( 'NONE',  ( 0.8660254037844394848, -0.4999999999999985012, 0.000000000000000000 ) ) ;
#5518=VERTEX_POINT ( 'NONE', #13579 ) ;
#5519=ADVANCED_FACE ( 'NONE', ( #24334 ), #13431, .F. ) ;
#5538=LINE ( 'NONE', #16195, #11127 ) ;
#5540=EDGE_CURVE ( 'NONE', #21098, #4583, #17873, .T. ) ;
#5542=DIRECTION ( 'NONE',  ( 0.2588190451025321748, 0.9659258262890653146, 0.000000000000000000 ) ) ;
#5547=DIRECTION ( 'NONE',  ( -0.000000000000000000, -0.000000000000000000, -1.000000000000000000 ) ) ;
#5550=PLANE ( 'NONE',  #25315 ) ;
#5560=VERTEX_POINT ( 'NONE', #5751 ) ;
#5567=DIRECTION ( 'NONE',  ( -0.000000000000000000, -0.000000000000000000, -1.000000000000000000 ) ) ;
#5571=DIRECTION ( 'NONE',  ( -0.4999999999999985012, -0.8660254037844394848, 0.000000000000000000 ) ) ;
#5580=EDGE_CURVE ( 'NONE', #7774, #962, #14661, .T. ) ;
#5583=DIRECTION ( 'NONE',  ( -0.9985600561963493549, -0.05364526231778204285, 0.000000000000000000 ) ) ;
#5628=EDGE_LOOP ( 'NONE', ( #14643, #11590, #24587, #20963 ) ) ;
#5636=ORIENTED_EDGE ( 'NONE', *, *, #4631, .T. ) ;
#5646=EDGE_LOOP ( 'NONE', ( #1267, #10214, #20044, #20218 ) ) ;
#5665=LINE ( 'NONE', #18874, #9919 ) ;
#5668=VERTEX_POINT ( 'NONE', #4010 ) ;
#5689=ORIENTED_EDGE ( 'NONE', *, *, #78, .F. ) ;
#5705=ORIENTED_EDGE ( 'NONE', *, *, #20182, .T. ) ;
#5709=CARTESIAN_POINT ( 'NONE',  ( 150.5563491861038870, 236.9705627484768797, -45.00000000000000000 ) ) ;
#5718=LINE ( 'NONE', #3554, #15761 ) ;
#5737=AXIS2_PLACEMENT_3D ( 'NONE', #28368, #26368, #19766 ) ;
#5738=VECTOR ( 'NONE', #14917, 999.9999999999998863 ) ;
#5742=ADVANCED_FACE ( 'NONE', ( #4303 ), #19959, .F. ) ;
#5751=CARTESIAN_POINT ( 'NONE',  ( 130.0130877889309602, 242.4751130497508029, -45.00000000000000000 ) ) ;
#5756=DIRECTION ( 'NONE',  ( 0.9659258262890670910, 0.2588190451025251804, 0.000000000000000000 ) ) ;
#5771=EDGE_LOOP ( 'NONE', ( #20927, #17595, #28024, #26444 ) ) ;
#5774=DIRECTION ( 'NONE',  ( -0.8916010070293515222, -0.4528218681382848443, 0.000000000000000000 ) ) ;
#5777=LINE ( 'NONE', #16563, #19054 ) ;
#5786=EDGE_CURVE ( 'NONE', #14926, #5668, #17372, .T. ) ;
#5819=PLANE ( 'NONE',  #16588 ) ;
#5831=EDGE_CURVE ( 'NONE', #22969, #10435, #25119, .T. ) ;
#5838=ADVANCED_FACE ( 'NONE', ( #13655 ), #5436, .F. ) ;
#5845=AXIS2_PLACEMENT_3D ( 'NONE', #8175, #23977, #4289 ) ;
#5854=DIRECTION ( 'NONE',  ( 0.4528218681382910060, 0.8916010070293484135, 0.000000000000000000 ) ) ;
#5867=EDGE_CURVE ( 'NONE', #25868, #13840, #13802, .T. ) ;
#5870=ORIENTED_EDGE ( 'NONE', *, *, #22190, .F. ) ;
#5873=LINE ( 'NONE', #25420, #6292 ) ;
#5885=CARTESIAN_POINT ( 'NONE',  ( 47.90501010967909679, 226.8374036014029969, 45.00000000000000000 ) ) ;
#5891=LINE ( 'NONE', #5470, #21534 ) ;
#5929=DIRECTION ( 'NONE',  ( -0.000000000000000000, -0.000000000000000000, -1.000000000000000000 ) ) ;
#5947=ORIENTED_EDGE ( 'NONE', *, *, #5242, .T. ) ;
#5965=DIRECTION ( 'NONE',  ( -0.7071067811865336949, 0.7071067811865614505, 0.000000000000000000 ) ) ;
#5980=VECTOR ( 'NONE', #1427, 1000.000000000000000 ) ;
#5983=ORIENTED_EDGE ( 'NONE', *, *, #9657, .T. ) ;
#5986=LINE ( 'NONE', #17467, #16048 ) ;
#5988=EDGE_CURVE ( 'NONE', #9639, #24350, #14778, .T. ) ;
#5991=DIRECTION ( 'NONE',  ( -0.000000000000000000, -0.000000000000000000, -1.000000000000000000 ) ) ;
#6007=EDGE_LOOP ( 'NONE', ( #1498, #6749, #25884, #9275 ) ) ;
#6015=VERTEX_POINT ( 'NONE', #10462 ) ;
#6016=ORIENTED_EDGE ( 'NONE', *, *, #17543, .F. ) ;
#6056=VECTOR ( 'NONE', #15141, 1000.000000000000000 ) ;
#6059=DIRECTION ( 'NONE',  ( -0.2588190451025252359, 0.9659258262890672020, 0.000000000000000000 ) ) ;
#6073=EDGE_CURVE ( 'NONE', #11332, #15143, #27400, .T. ) ;
#6076=CARTESIAN_POINT ( 'NONE',  ( 112.5248869502488134, 224.9869122110685282, 45.00000000000000000 ) ) ;
#6084=DIRECTION ( 'NONE',  ( -0.000000000000000000, -0.000000000000000000, -1.000000000000000000 ) ) ;
#6128=ORIENTED_EDGE ( 'NONE', *, *, #6236, .F. ) ;
#6134=VECTOR ( 'NONE', #8469, 1000.000000000000114 ) ;
#6137=EDGE_CURVE ( 'NONE', #11692, #22985, #10890, .T. ) ;
#6168=LINE ( 'NONE', #8753, #8751 ) ;
#6187=ORIENTED_EDGE ( 'NONE', *, *, #9397, .F. ) ;
#6216=LINE ( 'NONE', #6076, #9190 ) ;
#6236=EDGE_CURVE ( 'NONE', #14636, #23094, #2681, .T. ) ;
#6239=VECTOR ( 'NONE', #12407, 1000.000000000000000 ) ;
#6249=DIRECTION ( 'NONE',  ( -0.05364526231780537141, -0.9985600561963481336, 0.000000000000000000 ) ) ;
#6271=EDGE_CURVE ( 'NONE', #16518, #3496, #24377, .T. ) ;
#6292=VECTOR ( 'NONE', #1002, 1000.000000000000000 ) ;
#6305=PRODUCT_DEFINITION ( 'UNKNOWN', '', #22120, #18087 ) ;
#6308=VECTOR ( 'NONE', #20653, 1000.000000000000114 ) ;
#6348=CARTESIAN_POINT ( 'NONE',  ( 25.90578987075423001, -14.95671475544977724, 45.00000000000000000 ) ) ;
#6349=VERTEX_POINT ( 'NONE', #9588 ) ;
#6359=CARTESIAN_POINT ( 'NONE',  ( 162.6509609271901411, 34.34969631929494938, -45.00000000000000000 ) ) ;
#6362=ORIENTED_EDGE ( 'NONE', *, *, #17811, .F. ) ;
#6370=ORIENTED_EDGE ( 'NONE', *, *, #18268, .T. ) ;
#6375=EDGE_CURVE ( 'NONE', #5668, #10085, #16617, .T. ) ;
#6376=CARTESIAN_POINT ( 'NONE',  ( -40.00387671809203738, 149.2965004116384762, -45.00000000000000000 ) ) ;
#6378=LINE ( 'NONE', #26467, #27310 ) ;
#6388=DIRECTION ( 'NONE',  ( -0.7071067811865613395, -0.7071067811865335839, 0.000000000000000000 ) ) ;
#6403=LINE ( 'NONE', #10863, #6687 ) ;
#6411=EDGE_LOOP ( 'NONE', ( #1218, #9269, #21436, #4197 ) ) ;
#6413=DIRECTION ( 'NONE',  ( -0.000000000000000000, -0.000000000000000000, -1.000000000000000000 ) ) ;
#6452=ADVANCED_FACE ( 'NONE', ( #9864 ), #7712, .F. ) ;
#6475=DIRECTION ( 'NONE',  ( 0.9985600561963489108, -0.05364526231778980747, 0.000000000000000000 ) ) ;
#6479=ORIENTED_EDGE ( 'NONE', *, *, #17885, .T. ) ;
#6495=ORIENTED_EDGE ( 'NONE', *, *, #12897, .T. ) ;
#6501=ORIENTED_EDGE ( 'NONE', *, *, #3309, .F. ) ;
#6517=CARTESIAN_POINT ( 'NONE',  ( -41.54405845664282282, 46.26118624020713099, -45.00000000000000000 ) ) ;
#6519=DIRECTION ( 'NONE',  ( 0.5457381880580516320, -0.8379557447115657531, 0.000000000000000000 ) ) ;
#6530=PLANE ( 'NONE',  #15784 ) ;
#6540=VERTEX_POINT ( 'NONE', #12738 ) ;
#6579=LINE ( 'NONE', #24114, #10229 ) ;
#6582=ORIENTED_EDGE ( 'NONE', *, *, #12436, .T. ) ;
#6583=EDGE_LOOP ( 'NONE', ( #3421, #22094, #2246, #18460 ) ) ;
#6584=ORIENTED_EDGE ( 'NONE', *, *, #338, .F. ) ;
#6598=CARTESIAN_POINT ( 'NONE',  ( -26.22291647523108438, 23.54903675176048594, 45.00000000000000000 ) ) ;
#6610=PRODUCT ( 'Drive Gear', 'Drive Gear', '', ( #25859 ) ) ;
#6617=ADVANCED_FACE ( 'NONE', ( #26481 ), #788, .F. ) ;
#6632=VECTOR ( 'NONE', #20498, 1000.000000000000114 ) ;
#6646=VECTOR ( 'NONE', #3579, 1000.000000000000000 ) ;
#6663=DIRECTION ( 'NONE',  ( 0.3102637045530823312, 0.9506505318133460225, 0.000000000000000000 ) ) ;
#6676=EDGE_LOOP ( 'NONE', ( #18165, #8533, #14269, #7335 ) ) ;
#6680=CARTESIAN_POINT ( 'NONE',  ( 161.2365440327092472, 161.2365440327092472, -45.00000000000000000 ) ) ;
#6687=VECTOR ( 'NONE', #26075, 1000.000000000000114 ) ;
#6690=EDGE_CURVE ( 'NONE', #19703, #502, #13876, .T. ) ;
#6704=PLANE ( 'NONE',  #16669 ) ;
#6712=VERTEX_POINT ( 'NONE', #1345 ) ;
#6737=DIRECTION ( 'NONE',  ( 0.4528218681382909505, 0.8916010070293484135, -0.000000000000000000 ) ) ;
#6740=ORIENTED_EDGE ( 'NONE', *, *, #10198, .T. ) ;
#6749=ORIENTED_EDGE ( 'NONE', *, *, #6986, .F. ) ;
#6751=ORIENTED_EDGE ( 'NONE', *, *, #24894, .F. ) ;
#6756=EDGE_CURVE ( 'NONE', #28122, #7774, #16581, .T. ) ;
#6764=EDGE_CURVE ( 'NONE', #13241, #24120, #16444, .T. ) ;
#6768=CARTESIAN_POINT ( 'NONE',  ( 124.3660254037843771, 240.4185842870417105, 45.00000000000000000 ) ) ;
#6782=ADVANCED_FACE ( 'NONE', ( #25336 ), #7542, .F. ) ;
#6786=ORIENTED_EDGE ( 'NONE', *, *, #3300, .T. ) ;
#6794=VECTOR ( 'NONE', #5542, 999.9999999999998863 ) ;
#6799=CARTESIAN_POINT ( 'NONE',  ( -56.02075117275366978, 110.3042093914830559, 45.00000000000000000 ) ) ;
#6819=AXIS2_PLACEMENT_3D ( 'NONE', #20023, #4931, #2930 ) ;
#6828=EDGE_LOOP ( 'NONE', ( #11383, #5489, #16440, #23769 ) ) ;
#6840=CARTESIAN_POINT ( 'NONE',  ( 134.1167547769962596, -7.205103435269982093, 45.00000000000000000 ) ) ;
#6847=ORIENTED_EDGE ( 'NONE', *, *, #7733, .F. ) ;
#6852=LINE ( 'NONE', #5124, #6632 ) ;
#6864=EDGE_CURVE ( 'NONE', #9172, #4836, #6216, .T. ) ;
#6870=PLANE ( 'NONE',  #592 ) ;
#6876=PLANE ( 'NONE',  #26390 ) ;
#6896=EDGE_CURVE ( 'NONE', #3365, #23798, #10393, .T. ) ;
#6936=DIRECTION ( 'NONE',  ( -0.4528218681382693567, 0.8916010070293595158, 0.000000000000000000 ) ) ;
#6937=AXIS2_PLACEMENT_3D ( 'NONE', #23083, #16205, #25094 ) ;
#6950=ORIENTED_EDGE ( 'NONE', *, *, #11254, .F. ) ;
#6952=ORIENTED_EDGE ( 'NONE', *, *, #3439, .F. ) ;
#6961=ORIENTED_EDGE ( 'NONE', *, *, #27696, .T. ) ;
#6986=EDGE_CURVE ( 'NONE', #22985, #10405, #1152, .T. ) ;
#6992=ORIENTED_EDGE ( 'NONE', *, *, #5988, .T. ) ;
#7005=CARTESIAN_POINT ( 'NONE',  ( 3.660298066448477439, -2.383854334960948229, -45.00000000000000000 ) ) ;
#7029=FACE_OUTER_BOUND ( 'NONE', #28154, .T. ) ;
#7035=DIRECTION ( 'NONE',  ( -0.4999999999999985012, -0.8660254037844394848, 0.000000000000000000 ) ) ;
#7039=CARTESIAN_POINT ( 'NONE',  ( 133.9999999999998295, 242.9999999999997158, -45.00000000000000000 ) ) ;
#7040=CARTESIAN_POINT ( 'NONE',  ( 150.5563491861040575, 203.0294372515228929, -45.00000000000000000 ) ) ;
#7051=DIRECTION ( 'NONE',  ( -0.000000000000000000, -0.000000000000000000, -1.000000000000000000 ) ) ;
#7067=CARTESIAN_POINT ( 'NONE',  ( 176.1454027868280434, 57.48855481560072889, 45.00000000000000000 ) ) ;
#7069=LINE ( 'NONE', #884, #18335 ) ;
#7079=CARTESIAN_POINT ( 'NONE',  ( 216.4313787033304379, 124.9567147554451623, 45.00000000000000000 ) ) ;
#7084=DIRECTION ( 'NONE',  ( 0.05364526231776645809, -0.9985600561963501320, 0.000000000000000000 ) ) ;
#7088=AXIS2_PLACEMENT_3D ( 'NONE', #27511, #12033, #16344 ) ;
#7089=DIRECTION ( 'NONE',  ( -0.8916010070293484135, 0.4528218681382909505, 0.000000000000000000 ) ) ;
#7097=VERTEX_POINT ( 'NONE', #4146 ) ;
#7099=LINE ( 'NONE', #13721, #21009 ) ;
#7100=PLANE ( 'NONE',  #3744 ) ;
#7111=CARTESIAN_POINT ( 'NONE',  ( 136.0000000000000853, 196.9999999999997442, 45.00000000000000000 ) ) ;
#7120=VERTEX_POINT ( 'NONE', #26269 ) ;
#7139=CARTESIAN_POINT ( 'NONE',  ( 132.3894761555990556, 200.1711027725235397, 45.00000000000000000 ) ) ;
#7155=EDGE_CURVE ( 'NONE', #24989, #26858, #27988, .T. ) ;
#7156=EDGE_CURVE ( 'NONE', #3350, #627, #6168, .T. ) ;
#7160=CARTESIAN_POINT ( 'NONE',  ( 28.57744295357075259, -14.51376905457599342, 45.00000000000000000 ) ) ;
#7169=DIRECTION ( 'NONE',  ( 0.7440215159219069063, 0.6681556583950086781, 0.000000000000000000 ) ) ;
#7170=LINE ( 'NONE', #20234, #11297 ) ;
#7187=ORIENTED_EDGE ( 'NONE', *, *, #7657, .F. ) ;
#7199=CARTESIAN_POINT ( 'NONE',  ( 157.9999999999998579, 0.000000000000000000, 45.00000000000000000 ) ) ;
#7202=ORIENTED_EDGE ( 'NONE', *, *, #10850, .F. ) ;
#7203=DIRECTION ( 'NONE',  ( 0.000000000000000000, 1.000000000000000000, -0.000000000000000000 ) ) ;
#7216=DIRECTION ( 'NONE',  ( -0.000000000000000000, -0.000000000000000000, -1.000000000000000000 ) ) ;
#7232=PLANE ( 'NONE',  #17532 ) ;
#7233=ORIENTED_EDGE ( 'NONE', *, *, #3339, .T. ) ;
#7254=CARTESIAN_POINT ( 'NONE',  ( 135.9999999999998295, 242.9999999999997158, 45.00000000000000000 ) ) ;
#7266=EDGE_CURVE ( 'NONE', #24350, #28186, #4831, .T. ) ;
#7268=ORIENTED_EDGE ( 'NONE', *, *, #11735, .T. ) ;
#7283=LINE ( 'NONE', #20632, #4179 ) ;
#7287=CARTESIAN_POINT ( 'NONE',  ( 0.000000000000000000, 242.9999999999997158, -45.00000000000000000 ) ) ;
#7292=LINE ( 'NONE', #24670, #28166 ) ;
#7301=EDGE_LOOP ( 'NONE', ( #14233, #13066, #8994, #1209 ) ) ;
#7315=FACE_OUTER_BOUND ( 'NONE', #10046, .T. ) ;
#7335=ORIENTED_EDGE ( 'NONE', *, *, #4873, .T. ) ;
#7345=LINE ( 'NONE', #24864, #9157 ) ;
#7346=LINE ( 'NONE', #11375, #16490 ) ;
#7369=ORIENTED_EDGE ( 'NONE', *, *, #22916, .T. ) ;
#7387=AXIS2_PLACEMENT_3D ( 'NONE', #17129, #13121, #10811 ) ;
#7390=DIRECTION ( 'NONE',  ( -0.000000000000000000, -0.000000000000000000, -1.000000000000000000 ) ) ;
#7392=LINE ( 'NONE', #7670, #23488 ) ;
#7395=VERTEX_POINT ( 'NONE', #26959 ) ;
#7398=DIRECTION ( 'NONE',  ( 0.9506505318133482429, -0.3102637045530752258, 0.000000000000000000 ) ) ;
#7401=VECTOR ( 'NONE', #11942, 1000.000000000000000 ) ;
#7403=LINE ( 'NONE', #7111, #12475 ) ;
#7438=ORIENTED_EDGE ( 'NONE', *, *, #5988, .F. ) ;
#7442=EDGE_CURVE ( 'NONE', #860, #9208, #21154, .T. ) ;
#7447=VECTOR ( 'NONE', #4477, 999.9999999999998863 ) ;
#7451=MECHANICAL_DESIGN_GEOMETRIC_PRESENTATION_REPRESENTATION('',(#14790),#17091);
#7465=EDGE_CURVE ( 'NONE', #17680, #18077, #3343, .T. ) ;
#7474=VECTOR ( 'NONE', #3138, 999.9999999999998863 ) ;
#7486=EDGE_CURVE ( 'NONE', #2939, #15999, #25326, .T. ) ;
#7505=CARTESIAN_POINT ( 'NONE',  ( 11.56692809527929278, 215.3083398198040470, 45.00000000000000000 ) ) ;
#7509=EDGE_LOOP ( 'NONE', ( #5210, #24995, #6584, #5103 ) ) ;
#7520=LINE ( 'NONE', #5349, #11899 ) ;
#7536=FACE_OUTER_BOUND ( 'NONE', #12105, .T. ) ;
#7539=LINE ( 'NONE', #18587, #2230 ) ;
#7542=PLANE ( 'NONE',  #10557 ) ;
#7547=ORIENTED_EDGE ( 'NONE', *, *, #18693, .T. ) ;
#7561=ORIENTED_EDGE ( 'NONE', *, *, #17554, .F. ) ;
#7573=CARTESIAN_POINT ( 'NONE',  ( 111.9999999999999289, 218.9999999999996874, -45.00000000000000000 ) ) ;
#7579=EDGE_LOOP ( 'NONE', ( #25051, #8485, #26970, #15613 ) ) ;
#7594=ADVANCED_FACE ( 'NONE', ( #15274 ), #10527, .F. ) ;
#7599=CARTESIAN_POINT ( 'NONE',  ( 58.09044720719344213, 216.7965004116395562, 45.00000000000000000 ) ) ;
#7613=ORIENTED_EDGE ( 'NONE', *, *, #6756, .T. ) ;
#7648=ORIENTED_EDGE ( 'NONE', *, *, #10080, .T. ) ;
#7652=VERTEX_POINT ( 'NONE', #6768 ) ;
#7657=EDGE_CURVE ( 'NONE', #19790, #7652, #9514, .T. ) ;
#7660=VECTOR ( 'NONE', #12294, 1000.000000000000114 ) ;
#7662=PLANE ( 'NONE',  #14034 ) ;
#7670=CARTESIAN_POINT ( 'NONE',  ( 177.1897033089359184, 197.3087408678716770, 45.00000000000000000 ) ) ;
#7688=VERTEX_POINT ( 'NONE', #11537 ) ;
#7700=VECTOR ( 'NONE', #18641, 1000.000000000000114 ) ;
#7709=ORIENTED_EDGE ( 'NONE', *, *, #27755, .T. ) ;
#7712=PLANE ( 'NONE',  #15593 ) ;
#7721=ORIENTED_EDGE ( 'NONE', *, *, #19399, .T. ) ;
#7722=ORIENTED_EDGE ( 'NONE', *, *, #3717, .F. ) ;
#7725=EDGE_LOOP ( 'NONE', ( #20077, #6847, #6187, #26324 ) ) ;
#7733=EDGE_CURVE ( 'NONE', #9639, #14325, #18967, .T. ) ;
#7750=PLANE ( 'NONE',  #5166 ) ;
#7757=ORIENTED_EDGE ( 'NONE', *, *, #27019, .F. ) ;
#7760=CARTESIAN_POINT ( 'NONE',  ( 118.0294372515226939, 235.5563491861037164, -45.00000000000000000 ) ) ;
#7774=VERTEX_POINT ( 'NONE', #22997 ) ;
#7799=DIRECTION ( 'NONE',  ( 0.8660254037844394848, 0.4999999999999985012, -0.000000000000000000 ) ) ;
#7807=DIRECTION ( 'NONE',  ( -0.9784193629480828491, -0.2066290158914464437, 0.000000000000000000 ) ) ;
#7824=ORIENTED_EDGE ( 'NONE', *, *, #17747, .T. ) ;
#7838=CARTESIAN_POINT ( 'NONE',  ( 139.9869122110690114, 197.5248869502487139, -45.00000000000000000 ) ) ;
#7846=CARTESIAN_POINT ( 'NONE',  ( 114.5814157129579058, 230.6339745962151540, -45.00000000000000000 ) ) ;
#7864=VECTOR ( 'NONE', #5854, 1000.000000000000114 ) ;
#7878=DIRECTION ( 'NONE',  ( -0.000000000000000000, -0.000000000000000000, -1.000000000000000000 ) ) ;
#7883=LINE ( 'NONE', #20958, #16636 ) ;
#7905=VECTOR ( 'NONE', #13955, 999.9999999999998863 ) ;
#7917=VERTEX_POINT ( 'NONE', #8479 ) ;
#7936=DIRECTION ( 'NONE',  ( 0.9506505318133544602, 0.3102637045530566295, 0.000000000000000000 ) ) ;
#7959=CARTESIAN_POINT ( 'NONE',  ( 116.5224093497742786, 212.3463313526978595, 45.00000000000000000 ) ) ;
#7962=DIRECTION ( 'NONE',  ( -0.000000000000000000, -0.000000000000000000, -1.000000000000000000 ) ) ;
#7987=CARTESIAN_POINT ( 'NONE',  ( 155.4185842870420799, 209.3660254037844481, -45.00000000000000000 ) ) ;
#8011=VECTOR ( 'NONE', #14923, 1000.000000000000000 ) ;
#8012=CARTESIAN_POINT ( 'NONE',  ( -13.93137870332982331, 8.043285244550061108, -45.00000000000000000 ) ) ;
#8016=CARTESIAN_POINT ( 'NONE',  ( -41.04971513216914047, 194.3765543069588659, 45.00000000000000000 ) ) ;
#8018=FACE_OUTER_BOUND ( 'NONE', #27729, .T. ) ;
#8127=FACE_OUTER_BOUND ( 'NONE', #1765, .T. ) ;
#8134=EDGE_CURVE ( 'NONE', #11070, #11107, #26702, .T. ) ;
#8163=CARTESIAN_POINT ( 'NONE',  ( 185.9255560592262100, 121.0883471088020116, 45.00000000000000000 ) ) ;
#8168=EDGE_LOOP ( 'NONE', ( #641, #10959, #18737, #23162 ) ) ;
#8175=CARTESIAN_POINT ( 'NONE',  ( 134.9999999999998579, 220.0000000000000284, -45.00000000000000000 ) ) ;
#8180=DIRECTION ( 'NONE',  ( -0.000000000000000000, -0.000000000000000000, -1.000000000000000000 ) ) ;
#8181=EDGE_CURVE ( 'NONE', #21558, #4484, #11504, .T. ) ;
#8199=SHAPE_DEFINITION_REPRESENTATION ( #14625, #18912 ) ;
#8212=ORIENTED_EDGE ( 'NONE', *, *, #9091, .T. ) ;
#8216=LINE ( 'NONE', #3899, #10719 ) ;
#8230=LINE ( 'NONE', #8371, #196 ) ;
#8240=VERTEX_POINT ( 'NONE', #5159 ) ;
#8242=LINE ( 'NONE', #16999, #4656 ) ;
#8244=ORIENTED_EDGE ( 'NONE', *, *, #12160, .T. ) ;
#8248=ADVANCED_FACE ( 'NONE', ( #16237 ), #18241, .F. ) ;
#8253=ORIENTED_EDGE ( 'NONE', *, *, #7442, .F. ) ;
#8261=CARTESIAN_POINT ( 'NONE',  ( 114.5814157129578916, 209.3660254037841923, 45.00000000000000000 ) ) ;
#8275=CARTESIAN_POINT ( 'NONE',  ( 119.1329331941752230, 232.1752285801739220, -45.00000000000000000 ) ) ;
#8276=CARTESIAN_POINT ( 'NONE',  ( -36.37721155344281243, 172.2515494757248291, -45.00000000000000000 ) ) ;
#8279=FACE_OUTER_BOUND ( 'NONE', #1416, .T. ) ;
#8280=ORIENTED_EDGE ( 'NONE', *, *, #15265, .T. ) ;
#8281=DIRECTION ( 'NONE',  ( -1.000000000000000000, 0.000000000000000000, 0.000000000000000000 ) ) ;
#8289=VERTEX_POINT ( 'NONE', #3848 ) ;
#8292=DIRECTION ( 'NONE',  ( -0.000000000000000000, -0.000000000000000000, -1.000000000000000000 ) ) ;
#8318=ORIENTED_EDGE ( 'NONE', *, *, #21599, .F. ) ;
#8327=CARTESIAN_POINT ( 'NONE',  ( 118.0294372515226939, 235.5563491861037164, 45.00000000000000000 ) ) ;
#8336=LINE ( 'NONE', #14526, #25801 ) ;
#8349=CARTESIAN_POINT ( 'NONE',  ( 134.0000000000000853, 196.9999999999997442, -45.00000000000000000 ) ) ;
#8357=CARTESIAN_POINT ( 'NONE',  ( 156.9574749595459764, 213.0812361363529988, 45.00000000000000000 ) ) ;
#8363=VECTOR ( 'NONE', #23783, 1000.000000000000000 ) ;
#8367=ORIENTED_EDGE ( 'NONE', *, *, #27725, .T. ) ;
#8371=CARTESIAN_POINT ( 'NONE',  ( 124.9999999999998579, 220.0000000000000284, 45.00000000000000000 ) ) ;
#8393=LINE ( 'NONE', #17426, #20494 ) ;
#8406=ORIENTED_EDGE ( 'NONE', *, *, #13779, .F. ) ;
#8408=DIRECTION ( 'NONE',  ( 0.4528218681382693567, -0.8916010070293595158, 0.000000000000000000 ) ) ;
#8416=DIRECTION ( 'NONE',  ( 0.4999999999999985012, 0.8660254037844394848, -0.000000000000000000 ) ) ;
#8419=DIRECTION ( 'NONE',  ( -0.000000000000000000, 0.000000000000000000, 1.000000000000000000 ) ) ;
#8424=LINE ( 'NONE', #16762, #5183 ) ;
#8439=VECTOR ( 'NONE', #13009, 1000.000000000000000 ) ;
#8458=ORIENTED_EDGE ( 'NONE', *, *, #9301, .T. ) ;
#8463=ORIENTED_EDGE ( 'NONE', *, *, #16342, .T. ) ;
#8464=AXIS2_PLACEMENT_3D ( 'NONE', #23455, #12699, #10529 ) ;
#8468=LINE ( 'NONE', #15082, #2725 ) ;
#8469=DIRECTION ( 'NONE',  ( -0.7071067811865474617, -0.7071067811865474617, 0.000000000000000000 ) ) ;
#8479=CARTESIAN_POINT ( 'NONE',  ( 154.8288972274760908, 222.6105238444010297, 45.00000000000000000 ) ) ;
#8485=ORIENTED_EDGE ( 'NONE', *, *, #15234, .F. ) ;
#8495=AXIS2_PLACEMENT_3D ( 'NONE', #25518, #18772, #8281 ) ;
#8500=ORIENTED_EDGE ( 'NONE', *, *, #25628, .F. ) ;
#8516=CARTESIAN_POINT ( 'NONE',  ( -13.93137870332982331, 8.043285244550061108, 45.00000000000000000 ) ) ;
#8518=AXIS2_PLACEMENT_3D ( 'NONE', #4963, #13756, #22506 ) ;
#8525=ORIENTED_EDGE ( 'NONE', *, *, #21147, .T. ) ;
#8532=ADVANCED_FACE ( 'NONE', ( #27372 ), #9590, .F. ) ;
#8533=ORIENTED_EDGE ( 'NONE', *, *, #26710, .F. ) ;
#8543=DIRECTION ( 'NONE',  ( -0.4528218681383003319, -0.8916010070293436396, 0.000000000000000000 ) ) ;
#8562=ORIENTED_EDGE ( 'NONE', *, *, #27241, .F. ) ;
#8567=ORIENTED_EDGE ( 'NONE', *, *, #26142, .T. ) ;
#8580=AXIS2_PLACEMENT_3D ( 'NONE', #2471, #15006, #23755 ) ;
#8585=ADVANCED_FACE ( 'NONE', ( #9867, #18625 ), #5550, .F. ) ;
#8611=DIRECTION ( 'NONE',  ( -0.000000000000000000, -0.000000000000000000, -1.000000000000000000 ) ) ;
#8625=VERTEX_POINT ( 'NONE', #21059 ) ;
#8631=EDGE_LOOP ( 'NONE', ( #12437, #22640, #8849, #22868 ) ) ;
#8651=EDGE_CURVE ( 'NONE', #18634, #22236, #23502, .T. ) ;
#8652=EDGE_CURVE ( 'NONE', #15612, #19228, #19472, .T. ) ;
#8677=VERTEX_POINT ( 'NONE', #21480 ) ;
#8680=CARTESIAN_POINT ( 'NONE',  ( 162.0806940948679085, 180.4841764145329250, 45.00000000000000000 ) ) ;
#8682=LINE ( 'NONE', #1918, #14947 ) ;
#8711=ORIENTED_EDGE ( 'NONE', *, *, #13486, .T. ) ;
#8727=CARTESIAN_POINT ( 'NONE',  ( 151.9705627484769650, 235.5563491861038017, 45.00000000000000000 ) ) ;
#8751=VECTOR ( 'NONE', #14944, 1000.000000000000000 ) ;
#8753=CARTESIAN_POINT ( 'NONE',  ( 137.6105238444007455, 239.8288972274759203, 45.00000000000000000 ) ) ;
#8760=DIRECTION ( 'NONE',  ( -0.8916010070293484135, 0.4528218681382909505, 0.000000000000000000 ) ) ;
#8794=EDGE_CURVE ( 'NONE', #22498, #12331, #20033, .T. ) ;
#8795=LINE ( 'NONE', #22153, #26252 ) ;
#8833=DIRECTION ( 'NONE',  ( 0.8660254037844394848, -0.4999999999999985012, 0.000000000000000000 ) ) ;
#8849=ORIENTED_EDGE ( 'NONE', *, *, #19399, .F. ) ;
#8855=LINE ( 'NONE', #11308, #4357 ) ;
#8903=MANIFOLD_SOLID_BREP ( 'Boss-Extrude12', #14105 ) ;
#8908=CARTESIAN_POINT ( 'NONE',  ( 135.9999999999998295, 242.9999999999997158, 45.00000000000000000 ) ) ;
#8917=VERTEX_POINT ( 'NONE', #22906 ) ;
#8940=DIRECTION ( 'NONE',  ( -0.05364526231778202897, 0.9985600561963492439, 0.000000000000000000 ) ) ;
#8946=VECTOR ( 'NONE', #18677, 1000.000000000000000 ) ;
#8954=ORIENTED_EDGE ( 'NONE', *, *, #12561, .T. ) ;
#8977=CARTESIAN_POINT ( 'NONE',  ( 142.6536686473019699, 201.5224093497741649, 45.00000000000000000 ) ) ;
#8979=LINE ( 'NONE', #4511, #18593 ) ;
#8980=ORIENTED_EDGE ( 'NONE', *, *, #20287, .F. ) ;
#8991=EDGE_CURVE ( 'NONE', #3649, #28003, #1487, .T. ) ;
#8994=ORIENTED_EDGE ( 'NONE', *, *, #2234, .F. ) ;
#9009=DIRECTION ( 'NONE',  ( -0.2066290158914688702, -0.9784193629480781862, 0.000000000000000000 ) ) ;
#9062=VERTEX_POINT ( 'NONE', #25749 ) ;
#9081=AXIS2_PLACEMENT_3D ( 'NONE', #12062, #23110, #21368 ) ;
#9091=EDGE_CURVE ( 'NONE', #12262, #6349, #18870, .T. ) ;
#9101=LINE ( 'NONE', #22026, #10694 ) ;
#9117=AXIS2_PLACEMENT_3D ( 'NONE', #25926, #6249, #3524 ) ;
#9126=DIRECTION ( 'NONE',  ( -0.000000000000000000, -0.000000000000000000, -1.000000000000000000 ) ) ;
#9137=ORIENTED_EDGE ( 'NONE', *, *, #3666, .F. ) ;
#9141=VECTOR ( 'NONE', #20315, 999.9999999999998863 ) ;
#9150=CYLINDRICAL_SURFACE ( 'NONE', #8495, 10.00000000000000888 ) ;
#9154=VECTOR ( 'NONE', #24330, 1000.000000000000114 ) ;
#9157=VECTOR ( 'NONE', #13969, 1000.000000000000000 ) ;
#9166=CARTESIAN_POINT ( 'NONE',  ( -51.90955279280624524, 193.7290884209386661, -45.00000000000000000 ) ) ;
#9168=ORIENTED_EDGE ( 'NONE', *, *, #11735, .F. ) ;
#9172=VERTEX_POINT ( 'NONE', #9199 ) ;
#9174=CARTESIAN_POINT ( 'NONE',  ( 157.4751130497509450, 224.9869122110685566, -45.00000000000000000 ) ) ;
#9185=DIRECTION ( 'NONE',  ( -0.6681556583950127859, -0.7440215159219033536, 0.000000000000000000 ) ) ;
#9190=VECTOR ( 'NONE', #3915, 1000.000000000000000 ) ;
#9195=FACE_OUTER_BOUND ( 'NONE', #6583, .T. ) ;
#9196=ORIENTED_EDGE ( 'NONE', *, *, #14878, .T. ) ;
#9199=CARTESIAN_POINT ( 'NONE',  ( 112.5248869502488134, 224.9869122110685282, 45.00000000000000000 ) ) ;
#9201=VERTEX_POINT ( 'NONE', #17956 ) ;
#9208=VERTEX_POINT ( 'NONE', #7039 ) ;
#9214=CARTESIAN_POINT ( 'NONE',  ( 157.9999999999998579, 0.000000000000000000, -45.00000000000000000 ) ) ;
#9231=ORIENTED_EDGE ( 'NONE', *, *, #1466, .T. ) ;
#9244=VERTEX_POINT ( 'NONE', #16517 ) ;
#9255=LINE ( 'NONE', #2927, #13240 ) ;
#9269=ORIENTED_EDGE ( 'NONE', *, *, #15309, .F. ) ;
#9275=ORIENTED_EDGE ( 'NONE', *, *, #15309, .T. ) ;
#9276=CARTESIAN_POINT ( 'NONE',  ( 162.0806940948679085, 180.4841764145329250, -45.00000000000000000 ) ) ;
#9282=EDGE_LOOP ( 'NONE', ( #20896, #2792, #3965, #24796 ) ) ;
#9284=VECTOR ( 'NONE', #26889, 1000.000000000000114 ) ;
#9287=VECTOR ( 'NONE', #11884, 1000.000000000000000 ) ;
#9293=CARTESIAN_POINT ( 'NONE',  ( 111.5363082892543218, -5.992022692082500157, -45.00000000000000000 ) ) ;
#9301=EDGE_CURVE ( 'NONE', #28016, #22498, #1135, .T. ) ;
#9308=VECTOR ( 'NONE', #20390, 1000.000000000000000 ) ;
#9310=ORIENTED_EDGE ( 'NONE', *, *, #14238, .T. ) ;
#9322=ADVANCED_FACE ( 'NONE', ( #27407 ), #7750, .F. ) ;
#9338=CARTESIAN_POINT ( 'NONE',  ( 11.56692809527929278, 215.3083398198040470, 45.00000000000000000 ) ) ;
#9362=DIRECTION ( 'NONE',  ( -0.000000000000000000, -0.000000000000000000, -1.000000000000000000 ) ) ;
#9370=ORIENTED_EDGE ( 'NONE', *, *, #10835, .T. ) ;
#9377=DIRECTION ( 'NONE',  ( 0.6681556583950127859, 0.7440215159219033536, 0.000000000000000000 ) ) ;
#9378=EDGE_CURVE ( 'NONE', #14926, #18830, #7883, .T. ) ;
#9389=EDGE_CURVE ( 'NONE', #13728, #14325, #18945, .T. ) ;
#9397=EDGE_CURVE ( 'NONE', #5476, #9639, #27689, .T. ) ;
#9455=ORIENTED_EDGE ( 'NONE', *, *, #3406, .T. ) ;
#9465=EDGE_CURVE ( 'NONE', #4554, #5560, #6579, .T. ) ;
#9485=DIRECTION ( 'NONE',  ( -0.9985600561963492439, -0.05364526231778203591, 0.000000000000000000 ) ) ;
#9499=VERTEX_POINT ( 'NONE', #13919 ) ;
#9500=ORIENTED_EDGE ( 'NONE', *, *, #20647, .F. ) ;
#9505=CARTESIAN_POINT ( 'NONE',  ( 157.9999999999998579, 221.0000000000000284, 45.00000000000000000 ) ) ;
#9514=LINE ( 'NONE', #13396, #19309 ) ;
#9574=DIRECTION ( 'NONE',  ( 0.2066290158914672881, 0.9784193629480785193, 0.000000000000000000 ) ) ;
#9578=DIRECTION ( 'NONE',  ( -0.8916010070293515222, 0.4528218681382848443, 0.000000000000000000 ) ) ;
#9588=CARTESIAN_POINT ( 'NONE',  ( 116.5224093497742786, 212.3463313526978595, -45.00000000000000000 ) ) ;
#9590=PLANE ( 'NONE',  #6937 ) ;
#9591=ORIENTED_EDGE ( 'NONE', *, *, #12972, .F. ) ;
#9620=CARTESIAN_POINT ( 'NONE',  ( 176.5942101292460222, 101.9567147554491271, 45.00000000000000000 ) ) ;
#9623=EDGE_CURVE ( 'NONE', #15143, #4525, #16622, .T. ) ;
#9624=CARTESIAN_POINT ( 'NONE',  ( 176.1454027868280434, 57.48855481560072889, 45.00000000000000000 ) ) ;
#9639=VERTEX_POINT ( 'NONE', #15178 ) ;
#9650=ADVANCED_FACE ( 'NONE', ( #8279 ), #10434, .F. ) ;
#9654=LINE ( 'NONE', #5331, #17178 ) ;
#9657=EDGE_CURVE ( 'NONE', #7774, #12951, #8424, .T. ) ;
#9668=ORIENTED_EDGE ( 'NONE', *, *, #28147, .F. ) ;
#9689=LINE ( 'NONE', #5508, #2712 ) ;
#9719=LINE ( 'NONE', #9293, #22321 ) ;
#9726=VERTEX_POINT ( 'NONE', #21483 ) ;
#9739=ORIENTED_EDGE ( 'NONE', *, *, #1216, .F. ) ;
#9741=ORIENTED_EDGE ( 'NONE', *, *, #15800, .T. ) ;
#9776=ORIENTED_EDGE ( 'NONE', *, *, #3052, .F. ) ;
#9777=LINE ( 'NONE', #18535, #17020 ) ;
#9792=DIRECTION ( 'NONE',  ( -0.000000000000000000, -0.000000000000000000, -1.000000000000000000 ) ) ;
#9799=CARTESIAN_POINT ( 'NONE',  ( -36.37721155344281243, 172.2515494757248291, 45.00000000000000000 ) ) ;
#9817=PLANE ( 'NONE',  #4851 ) ;
#9837=ORIENTED_EDGE ( 'NONE', *, *, #6764, .T. ) ;
#9838=VECTOR ( 'NONE', #5424, 1000.000000000000227 ) ;
#9847=ORIENTED_EDGE ( 'NONE', *, *, #6896, .F. ) ;
#9848=ORIENTED_EDGE ( 'NONE', *, *, #21293, .F. ) ;
#9850=EDGE_CURVE ( 'NONE', #3329, #21558, #11292, .T. ) ;
#9855=PLANE ( 'NONE',  #8518 ) ;
#9864=FACE_OUTER_BOUND ( 'NONE', #18627, .T. ) ;
#9865=DIRECTION ( 'NONE',  ( -0.000000000000000000, -0.000000000000000000, -1.000000000000000000 ) ) ;
#9867=FACE_BOUND ( 'NONE', #1974, .T. ) ;
#9881=ORIENTED_EDGE ( 'NONE', *, *, #21508, .F. ) ;
#9889=CARTESIAN_POINT ( 'NONE',  ( 122.8247714198253959, 235.8670668058242939, -45.00000000000000000 ) ) ;
#9906=ORIENTED_EDGE ( 'NONE', *, *, #20620, .F. ) ;
#9912=ORIENTED_EDGE ( 'NONE', *, *, #11402, .F. ) ;
#9919=VECTOR ( 'NONE', #7962, 1000.000000000000000 ) ;
#9933=DIRECTION ( 'NONE',  ( -0.000000000000000000, -0.000000000000000000, -1.000000000000000000 ) ) ;
#9953=FACE_OUTER_BOUND ( 'NONE', #18864, .T. ) ;
#9955=DIRECTION ( 'NONE',  ( -0.6681556583950251094, -0.7440215159218921404, 0.000000000000000000 ) ) ;
#9967=ORIENTED_EDGE ( 'NONE', *, *, #8991, .T. ) ;
#10001=CARTESIAN_POINT ( 'NONE',  ( 128.0812361363530272, 198.0425250404537394, 45.00000000000000000 ) ) ;
#10015=DIRECTION ( 'NONE',  ( 0.8379557447115549840, 0.5457381880580680633, 0.000000000000000000 ) ) ;
#10023=CARTESIAN_POINT ( 'NONE',  ( 151.9705627484771355, 204.4436508138959141, -45.00000000000000000 ) ) ;
#10046=EDGE_LOOP ( 'NONE', ( #25832, #145, #17536, #8367 ) ) ;
#10080=EDGE_CURVE ( 'NONE', #22485, #4554, #8242, .T. ) ;
#10083=VECTOR ( 'NONE', #21731, 1000.000000000000000 ) ;
#10085=VERTEX_POINT ( 'NONE', #23468 ) ;
#10094=FACE_OUTER_BOUND ( 'NONE', #11068, .T. ) ;
#10095=CARTESIAN_POINT ( 'NONE',  ( -54.22951502486254327, 83.26691194124390449, 45.00000000000000000 ) ) ;
#10101=LINE ( 'NONE', #14844, #21142 ) ;
#10128=EDGE_LOOP ( 'NONE', ( #20785, #13926, #404, #24430 ) ) ;
#10137=EDGE_CURVE ( 'NONE', #18830, #10085, #15709, .T. ) ;
#10139=CARTESIAN_POINT ( 'NONE',  ( 127.3463313526982716, 201.5224093497739943, -45.00000000000000000 ) ) ;
#10141=EDGE_CURVE ( 'NONE', #2873, #18634, #4343, .T. ) ;
#10156=VERTEX_POINT ( 'NONE', #2612 ) ;
#10157=LINE ( 'NONE', #1388, #22734 ) ;
#10178=PLANE ( 'NONE',  #9081 ) ;
#10186=CARTESIAN_POINT ( 'NONE',  ( -12.00299901279919723, 223.4254219457707222, -45.00000000000000000 ) ) ;
#10195=ORIENTED_EDGE ( 'NONE', *, *, #21022, .T. ) ;
#10198=EDGE_CURVE ( 'NONE', #2939, #19703, #17422, .T. ) ;
#10214=ORIENTED_EDGE ( 'NONE', *, *, #12857, .F. ) ;
#10229=VECTOR ( 'NONE', #11036, 1000.000000000000114 ) ;
#10233=EDGE_LOOP ( 'NONE', ( #13581, #13118, #6582, #24032 ) ) ;
#10236=CARTESIAN_POINT ( 'NONE',  ( 132.3894761555988282, 239.8288972274758919, 45.00000000000000000 ) ) ;
#10239=LINE ( 'NONE', #23169, #6239 ) ;
#10242=EDGE_CURVE ( 'NONE', #6712, #22236, #42, .T. ) ;
#10247=CARTESIAN_POINT ( 'NONE',  ( -41.04971513216914047, 194.3765543069588659, -45.00000000000000000 ) ) ;
#10263=ORIENTED_EDGE ( 'NONE', *, *, #3005, .F. ) ;
#10269=VECTOR ( 'NONE', #8940, 1000.000000000000227 ) ;
#10285=VERTEX_POINT ( 'NONE', #15563 ) ;
#10291=VECTOR ( 'NONE', #14562, 1000.000000000000114 ) ;
#10293=ORIENTED_EDGE ( 'NONE', *, *, #20668, .T. ) ;
#10375=CARTESIAN_POINT ( 'NONE',  ( -40.00387671809203738, 149.2965004116384762, 45.00000000000000000 ) ) ;
#10393=LINE ( 'NONE', #12704, #26154 ) ;
#10402=VECTOR ( 'NONE', #13600, 1000.000000000000000 ) ;
#10405=VERTEX_POINT ( 'NONE', #8349 ) ;
#10425=ORIENTED_EDGE ( 'NONE', *, *, #78, .T. ) ;
#10434=PLANE ( 'NONE',  #1976 ) ;
#10435=VERTEX_POINT ( 'NONE', #16965 ) ;
#10436=DIRECTION ( 'NONE',  ( -0.2066290158914672603, -0.9784193629480785193, 0.000000000000000000 ) ) ;
#10441=VERTEX_POINT ( 'NONE', #3885 ) ;
#10449=FACE_OUTER_BOUND ( 'NONE', #13989, .T. ) ;
#10452=CARTESIAN_POINT ( 'NONE',  ( 155.4185842870419947, 230.6339745962152392, 45.00000000000000000 ) ) ;
#10462=CARTESIAN_POINT ( 'NONE',  ( 118.0294372515228787, 204.4436508138956015, -45.00000000000000000 ) ) ;
#10473=VERTEX_POINT ( 'NONE', #21983 ) ;
#10494=ORIENTED_EDGE ( 'NONE', *, *, #338, .T. ) ;
#10501=ORIENTED_EDGE ( 'NONE', *, *, #16374, .T. ) ;
#10516=PLANE ( 'NONE',  #4269 ) ;
#10527=PLANE ( 'NONE',  #7387 ) ;
#10529=DIRECTION ( 'NONE',  ( -0.9506505318133544602, -0.3102637045530566295, 0.000000000000000000 ) ) ;
#10542=ORIENTED_EDGE ( 'NONE', *, *, #26928, .T. ) ;
#10557=AXIS2_PLACEMENT_3D ( 'NONE', #27475, #16859, #16722 ) ;
#10566=FACE_OUTER_BOUND ( 'NONE', #40, .T. ) ;
#10603=ADVANCED_FACE ( 'NONE', ( #5311 ), #27004, .F. ) ;
#10605=CARTESIAN_POINT ( 'NONE',  ( 145.6339745962156940, 199.5814157129578064, 45.00000000000000000 ) ) ;
#10613=ORIENTED_EDGE ( 'NONE', *, *, #20620, .T. ) ;
#10637=AXIS2_PLACEMENT_3D ( 'NONE', #25065, #2320, #14860 ) ;
#10646=CARTESIAN_POINT ( 'NONE',  ( -56.02075117275366978, 110.3042093914830559, -45.00000000000000000 ) ) ;
#10694=VECTOR ( 'NONE', #6936, 999.9999999999998863 ) ;
#10712=LINE ( 'NONE', #3811, #11429 ) ;
#10719=VECTOR ( 'NONE', #2447, 1000.000000000000114 ) ;
#10728=VERTEX_POINT ( 'NONE', #24095 ) ;
#10746=CARTESIAN_POINT ( 'NONE',  ( 128.0812361363530272, 198.0425250404537394, -45.00000000000000000 ) ) ;
#10758=ORIENTED_EDGE ( 'NONE', *, *, #22790, .T. ) ;
#10762=ORIENTED_EDGE ( 'NONE', *, *, #12650, .F. ) ;
#10772=DIRECTION ( 'NONE',  ( 0.9985600561963501320, 0.05364526231776645809, -0.000000000000000000 ) ) ;
#10781=AXIS2_PLACEMENT_3D ( 'NONE', #21587, #17139, #1897 ) ;
#10782=ORIENTED_EDGE ( 'NONE', *, *, #18268, .F. ) ;
#10811=DIRECTION ( 'NONE',  ( 0.2066290158914390052, -0.9784193629480844034, 0.000000000000000000 ) ) ;
#10830=VECTOR ( 'NONE', #12200, 1000.000000000000000 ) ;
#10835=EDGE_CURVE ( 'NONE', #23798, #9201, #24660, .T. ) ;
#10839=AXIS2_PLACEMENT_3D ( 'NONE', #18577, #20870, #20724 ) ;
#10850=EDGE_CURVE ( 'NONE', #7120, #3880, #5538, .T. ) ;
#10859=ORIENTED_EDGE ( 'NONE', *, *, #27421, .T. ) ;
#10863=CARTESIAN_POINT ( 'NONE',  ( 175.6862808370088089, 157.7720269260891826, 45.00000000000000000 ) ) ;
#10872=CARTESIAN_POINT ( 'NONE',  ( 147.3660254037845334, 200.5814157129577779, 45.00000000000000000 ) ) ;
#10873=FACE_OUTER_BOUND ( 'NONE', #5771, .T. ) ;
#10885=CARTESIAN_POINT ( 'NONE',  ( 112.5248869502488134, 224.9869122110685282, -45.00000000000000000 ) ) ;
#10890=LINE ( 'NONE', #4274, #3640 ) ;
#10922=EDGE_CURVE ( 'NONE', #26795, #6015, #14312, .T. ) ;
#10954=CARTESIAN_POINT ( 'NONE',  ( 157.4751130497510303, 215.0130877889310455, 45.00000000000000000 ) ) ;
#10959=ORIENTED_EDGE ( 'NONE', *, *, #8794, .F. ) ;
#10963=VECTOR ( 'NONE', #27849, 1000.000000000000000 ) ;
#10981=LINE ( 'NONE', #22032, #26410 ) ;
#10996=LINE ( 'NONE', #16580, #14375 ) ;
#11007=ORIENTED_EDGE ( 'NONE', *, *, #20546, .T. ) ;
#11015=EDGE_CURVE ( 'NONE', #10405, #4982, #16674, .T. ) ;
#11018=PLANE ( 'NONE',  #5737 ) ;
#11036=DIRECTION ( 'NONE',  ( -0.6681556583950049033, 0.7440215159219103480, 0.000000000000000000 ) ) ;
#11060=VECTOR ( 'NONE', #14235, 1000.000000000000227 ) ;
#11068=EDGE_LOOP ( 'NONE', ( #2910, #27618, #7722, #5705 ) ) ;
#11070=VERTEX_POINT ( 'NONE', #19387 ) ;
#11097=CARTESIAN_POINT ( 'NONE',  ( 154.4185842870420799, 207.6339745962155803, -45.00000000000000000 ) ) ;
#11098=DIRECTION ( 'NONE',  ( -0.4999999999999865108, 0.8660254037844464792, 0.000000000000000000 ) ) ;
#11103=CARTESIAN_POINT ( 'NONE',  ( 204.8742559748123426, 133.4291290931197977, 45.00000000000000000 ) ) ;
#11107=VERTEX_POINT ( 'NONE', #12935 ) ;
#11113=FACE_OUTER_BOUND ( 'NONE', #340, .T. ) ;
#11127=VECTOR ( 'NONE', #9578, 1000.000000000000114 ) ;
#11133=VECTOR ( 'NONE', #23258, 999.9999999999998863 ) ;
#11140=ORIENTED_EDGE ( 'NONE', *, *, #23931, .F. ) ;
#11144=CARTESIAN_POINT ( 'NONE',  ( 147.3660254037842492, 239.4185842870417673, 45.00000000000000000 ) ) ;
#11167=VERTEX_POINT ( 'NONE', #17089 ) ;
#11170=VECTOR ( 'NONE', #8833, 1000.000000000000114 ) ;
#11172=FACE_OUTER_BOUND ( 'NONE', #25266, .T. ) ;
#11189=VECTOR ( 'NONE', #7084, 1000.000000000000114 ) ;
#11191=VECTOR ( 'NONE', #3063, 1000.000000000000114 ) ;
#11220=ORIENTED_EDGE ( 'NONE', *, *, #5214, .F. ) ;
#11228=ADVANCED_BREP_SHAPE_REPRESENTATION ( '', ( #8903, #10637 ), #19371 ) ;
#11230=AXIS2_PLACEMENT_3D ( 'NONE', #16291, #7799, #20869 ) ;
#11245=ADVANCED_FACE ( 'NONE', ( #7029 ), #24555, .F. ) ;
#11254=EDGE_CURVE ( 'NONE', #14719, #21880, #12487, .T. ) ;
#11267=CARTESIAN_POINT ( 'NONE',  ( 48.74042075079900371, -13.05995637893015449, -45.00000000000000000 ) ) ;
#11270=DIRECTION ( 'NONE',  ( -0.000000000000000000, -0.000000000000000000, -1.000000000000000000 ) ) ;
#11292=LINE ( 'NONE', #15895, #16214 ) ;
#11294=ADVANCED_FACE ( 'NONE', ( #8018 ), #16785, .F. ) ;
#11297=VECTOR ( 'NONE', #15943, 1000.000000000000114 ) ;
#11308=CARTESIAN_POINT ( 'NONE',  ( -26.22291647523108438, 23.54903675176048594, 45.00000000000000000 ) ) ;
#11330=VERTEX_POINT ( 'NONE', #25259 ) ;
#11332=VERTEX_POINT ( 'NONE', #27820 ) ;
#11355=CARTESIAN_POINT ( 'NONE',  ( -56.65306767071049165, 63.08575069354419185, 45.00000000000000000 ) ) ;
#11375=CARTESIAN_POINT ( 'NONE',  ( 157.9999999999998579, 221.0000000000000284, 45.00000000000000000 ) ) ;
#11383=ORIENTED_EDGE ( 'NONE', *, *, #10141, .T. ) ;
#11387=LINE ( 'NONE', #324, #1118 ) ;
#11398=DIRECTION ( 'NONE',  ( -0.8660254037844464792, -0.4999999999999865108, 0.000000000000000000 ) ) ;
#11402=EDGE_CURVE ( 'NONE', #14035, #194, #5718, .T. ) ;
#11413=VECTOR ( 'NONE', #12479, 1000.000000000000114 ) ;
#11417=CARTESIAN_POINT ( 'NONE',  ( 150.8670668058247202, 207.8247714198255949, 45.00000000000000000 ) ) ;
#11425=CARTESIAN_POINT ( 'NONE',  ( 139.9869122110690114, 197.5248869502487139, 45.00000000000000000 ) ) ;
#11429=VECTOR ( 'NONE', #21617, 1000.000000000000000 ) ;
#11430=DIRECTION ( 'NONE',  ( 0.9659258262890705327, 0.2588190451025121908, 0.000000000000000000 ) ) ;
#11450=ORIENTED_EDGE ( 'NONE', *, *, #5867, .F. ) ;
#11455=VECTOR ( 'NONE', #11837, 999.9999999999998863 ) ;
#11484=LINE ( 'NONE', #18640, #12287 ) ;
#11504=LINE ( 'NONE', #20244, #1887 ) ;
#11512=EDGE_LOOP ( 'NONE', ( #15010, #24645, #8406, #25710 ) ) ;
#11519=ORIENTED_EDGE ( 'NONE', *, *, #27281, .T. ) ;
#11537=CARTESIAN_POINT ( 'NONE',  ( 137.6105238444012286, 200.1711027725236534, 45.00000000000000000 ) ) ;
#11554=AXIS2_PLACEMENT_3D ( 'NONE', #8016, #1551, #23672 ) ;
#11582=( LENGTH_UNIT ( ) NAMED_UNIT ( * ) SI_UNIT ( .MILLI., .METRE. ) );
#11590=ORIENTED_EDGE ( 'NONE', *, *, #10242, .F. ) ;
#11602=CARTESIAN_POINT ( 'NONE',  ( 95.82124051657368113, -20.23615780638419182, 45.00000000000000000 ) ) ;
#11615=EDGE_CURVE ( 'NONE', #962, #11738, #24522, .T. ) ;
#11617=CARTESIAN_POINT ( 'NONE',  ( -15.28840184913744515, 9.956927649352207865, 45.00000000000000000 ) ) ;
#11618=VECTOR ( 'NONE', #2988, 1000.000000000000000 ) ;
#11620=ORIENTED_EDGE ( 'NONE', *, *, #13063, .T. ) ;
#11628=ADVANCED_FACE ( 'NONE', ( #22658 ), #2817, .F. ) ;
#11630=ORIENTED_EDGE ( 'NONE', *, *, #24053, .T. ) ;
#11638=LINE ( 'NONE', #1259, #21265 ) ;
#11639=CARTESIAN_POINT ( 'NONE',  ( 111.3836151241014960, 219.3130464734738325, 45.00000000000000000 ) ) ;
#11692=VERTEX_POINT ( 'NONE', #7139 ) ;
#11707=ADVANCED_FACE ( 'NONE', ( #4542 ), #6704, .F. ) ;
#11710=ORIENTED_EDGE ( 'NONE', *, *, #27121, .F. ) ;
#11716=CARTESIAN_POINT ( 'NONE',  ( -13.93137870332982331, 8.043285244550061108, 45.00000000000000000 ) ) ;
#11721=LINE ( 'NONE', #7254, #18043 ) ;
#11723=LINE ( 'NONE', #18030, #18124 ) ;
#11731=VERTEX_POINT ( 'NONE', #16612 ) ;
#11735=EDGE_CURVE ( 'NONE', #14223, #9726, #16753, .T. ) ;
#11738=VERTEX_POINT ( 'NONE', #10001 ) ;
#11762=AXIS2_PLACEMENT_3D ( 'NONE', #27518, #1666, #10436 ) ;
#11794=ORIENTED_EDGE ( 'NONE', *, *, #6271, .F. ) ;
#11837=DIRECTION ( 'NONE',  ( 0.9506505318133544602, 0.3102637045530566295, 0.000000000000000000 ) ) ;
#11846=CARTESIAN_POINT ( 'NONE',  ( 142.6536686473015152, 238.4775906502254941, 45.00000000000000000 ) ) ;
#11849=ADVANCED_FACE ( 'NONE', ( #27096 ), #23352, .F. ) ;
#11850=CARTESIAN_POINT ( 'NONE',  ( 127.3463313526982716, 201.5224093497739943, 45.00000000000000000 ) ) ;
#11860=DIRECTION ( 'NONE',  ( 0.7440215159218921404, -0.6681556583950252204, 0.000000000000000000 ) ) ;
#11861=( NAMED_UNIT ( * ) PLANE_ANGLE_UNIT ( ) SI_UNIT ( $, .RADIAN. ) );
#11869=ORIENTED_EDGE ( 'NONE', *, *, #13669, .T. ) ;
#11870=EDGE_CURVE ( 'NONE', #4776, #9726, #23774, .T. ) ;
#11874=AXIS2_PLACEMENT_3D ( 'NONE', #14698, #5504, #3342 ) ;
#11884=DIRECTION ( 'NONE',  ( 0.7071067811865613395, 0.7071067811865336949, 0.000000000000000000 ) ) ;
#11886=CARTESIAN_POINT ( 'NONE',  ( 58.09044720719344213, 216.7965004116395562, 45.00000000000000000 ) ) ;
#11899=VECTOR ( 'NONE', #1318, 999.9999999999998863 ) ;
#11903=ADVANCED_FACE ( 'NONE', ( #17302 ), #6530, .F. ) ;
#11910=ORIENTED_EDGE ( 'NONE', *, *, #24532, .T. ) ;
#11926=VECTOR ( 'NONE', #7203, 1000.000000000000000 ) ;
#11942=DIRECTION ( 'NONE',  ( 0.000000000000000000, 1.000000000000000000, -0.000000000000000000 ) ) ;
#11974=DIRECTION ( 'NONE',  ( 0.8379557447115515423, -0.5457381880580733924, 0.000000000000000000 ) ) ;
#12005=ORIENTED_EDGE ( 'NONE', *, *, #5266, .T. ) ;
#12006=ORIENTED_EDGE ( 'NONE', *, *, #14096, .F. ) ;
#12033=DIRECTION ( 'NONE',  ( -0.5457381880580733924, -0.8379557447115515423, 0.000000000000000000 ) ) ;
#12037=ORIENTED_EDGE ( 'NONE', *, *, #14838, .T. ) ;
#12056=CARTESIAN_POINT ( 'NONE',  ( 113.0425250404539241, 213.0812361363525440, 45.00000000000000000 ) ) ;
#12060=EDGE_CURVE ( 'NONE', #9244, #18948, #15883, .T. ) ;
#12062=CARTESIAN_POINT ( 'NONE',  ( -66.26041567618258910, 130.4659900502583127, 45.00000000000000000 ) ) ;
#12065=VECTOR ( 'NONE', #557, 1000.000000000000114 ) ;
#12083=AXIS2_PLACEMENT_3D ( 'NONE', #4937, #26348, #11430 ) ;
#12090=LINE ( 'NONE', #740, #8946 ) ;
#12100=CARTESIAN_POINT ( 'NONE',  ( 134.1167547769962596, -7.205103435269982093, 45.00000000000000000 ) ) ;
#12105=EDGE_LOOP ( 'NONE', ( #11910, #4231, #12955, #24887 ) ) ;
#12140=ORIENTED_EDGE ( 'NONE', *, *, #9465, .T. ) ;
#12155=CARTESIAN_POINT ( 'NONE',  ( 140.5127944162910865, 243.3752990424897575, 45.00000000000000000 ) ) ;
#12160=EDGE_CURVE ( 'NONE', #14719, #20334, #27469, .T. ) ;
#12165=LINE ( 'NONE', #3091, #23200 ) ;
#12200=DIRECTION ( 'NONE',  ( -0.000000000000000000, -0.000000000000000000, -1.000000000000000000 ) ) ;
#12208=VECTOR ( 'NONE', #20989, 1000.000000000000000 ) ;
#12218=DIRECTION ( 'NONE',  ( 0.05364526231779760679, -0.9985600561963485777, 0.000000000000000000 ) ) ;
#12232=VECTOR ( 'NONE', #9955, 1000.000000000000114 ) ;
#12233=CARTESIAN_POINT ( 'NONE',  ( 122.8247714198256944, 204.1329331941749672, 45.00000000000000000 ) ) ;
#12244=DIRECTION ( 'NONE',  ( -0.2066290158914539099, 0.9784193629480814058, 0.000000000000000000 ) ) ;
#12259=DIRECTION ( 'NONE',  ( 1.000000000000000000, -1.387778780781444413E-14, 0.000000000000000000 ) ) ;
#12262=VERTEX_POINT ( 'NONE', #27332 ) ;
#12267=CARTESIAN_POINT ( 'NONE',  ( 150.8670668058245212, 232.1752285801742630, -45.00000000000000000 ) ) ;
#12287=VECTOR ( 'NONE', #16078, 1000.000000000000000 ) ;
#12294=DIRECTION ( 'NONE',  ( 0.4999999999999985012, 0.8660254037844394848, 0.000000000000000000 ) ) ;
#12323=ORIENTED_EDGE ( 'NONE', *, *, #14096, .T. ) ;
#12324=FACE_OUTER_BOUND ( 'NONE', #21236, .T. ) ;
#12331=VERTEX_POINT ( 'NONE', #12980 ) ;
#12350=EDGE_LOOP ( 'NONE', ( #15995, #9137, #23608, #26395 ) ) ;
#12352=EDGE_CURVE ( 'NONE', #10435, #2939, #21298, .T. ) ;
#12357=ORIENTED_EDGE ( 'NONE', *, *, #8991, .F. ) ;
#12367=ADVANCED_FACE ( 'NONE', ( #23317 ), #21156, .F. ) ;
#12369=LINE ( 'NONE', #21107, #24023 ) ;
#12378=LINE ( 'NONE', #5885, #10963 ) ;
#12379=CARTESIAN_POINT ( 'NONE',  ( -54.22951502486254327, 83.26691194124390449, 45.00000000000000000 ) ) ;
#12391=ORIENTED_EDGE ( 'NONE', *, *, #10137, .F. ) ;
#12393=VECTOR ( 'NONE', #7216, 1000.000000000000000 ) ;
#12407=DIRECTION ( 'NONE',  ( -0.000000000000000000, -0.000000000000000000, -1.000000000000000000 ) ) ;
#12409=DIRECTION ( 'NONE',  ( 0.6681556583950049033, -0.7440215159219103480, 0.000000000000000000 ) ) ;
#12411=ORIENTED_EDGE ( 'NONE', *, *, #22501, .F. ) ;
#12434=ORIENTED_EDGE ( 'NONE', *, *, #26038, .F. ) ;
#12436=EDGE_CURVE ( 'NONE', #24234, #16719, #8230, .T. ) ;
#12437=ORIENTED_EDGE ( 'NONE', *, *, #13405, .T. ) ;
#12441=ADVANCED_FACE ( 'NONE', ( #17133 ), #25889, .F. ) ;
#12456=CARTESIAN_POINT ( 'NONE',  ( 117.5127944162877753, 203.5381304684075019, 45.00000000000000000 ) ) ;
#12464=CARTESIAN_POINT ( 'NONE',  ( 144.9999999999998863, 220.0000000000000284, 45.00000000000000000 ) ) ;
#12475=VECTOR ( 'NONE', #2940, 1000.000000000000000 ) ;
#12479=DIRECTION ( 'NONE',  ( -0.2066290158914389774, 0.9784193629480844034, 0.000000000000000000 ) ) ;
#12486=FACE_OUTER_BOUND ( 'NONE', #7579, .T. ) ;
#12487=LINE ( 'NONE', #14632, #4697 ) ;
#12488=ORIENTED_EDGE ( 'NONE', *, *, #27421, .F. ) ;
#12503=CARTESIAN_POINT ( 'NONE',  ( 118.0294372515228787, 204.4436508138956015, 45.00000000000000000 ) ) ;
#12510=CARTESIAN_POINT ( 'NONE',  ( 142.6536686473015152, 238.4775906502254941, 45.00000000000000000 ) ) ;
#12521=EDGE_CURVE ( 'NONE', #24989, #3649, #2746, .T. ) ;
#12546=PLANE ( 'NONE',  #27708 ) ;
#12561=EDGE_CURVE ( 'NONE', #20475, #10473, #11387, .T. ) ;
#12592=DIRECTION ( 'NONE',  ( 0.7440215159218956931, -0.6681556583950213346, 0.000000000000000000 ) ) ;
#12601=DIRECTION ( 'NONE',  ( 0.9784193629480814058, 0.2066290158914539099, 0.000000000000000000 ) ) ;
#12615=LINE ( 'NONE', #16286, #11455 ) ;
#12617=EDGE_CURVE ( 'NONE', #20334, #23507, #4759, .T. ) ;
#12644=EDGE_CURVE ( 'NONE', #22485, #13260, #9654, .T. ) ;
#12649=DIRECTION ( 'NONE',  ( 0.9985600561963492439, 0.05364526231778202897, 0.000000000000000000 ) ) ;
#12650=EDGE_CURVE ( 'NONE', #10435, #20930, #5190, .T. ) ;
#12670=EDGE_CURVE ( 'NONE', #22498, #24909, #24740, .T. ) ;
#12677=CARTESIAN_POINT ( 'NONE',  ( 11.56692809527929278, 215.3083398198040470, -45.00000000000000000 ) ) ;
#12687=DIRECTION ( 'NONE',  ( -0.4528218681382848443, 0.8916010070293515222, 0.000000000000000000 ) ) ;
#12699=DIRECTION ( 'NONE',  ( -0.3102637045530566295, 0.9506505318133544602, 0.000000000000000000 ) ) ;
#12704=CARTESIAN_POINT ( 'NONE',  ( 74.37710191228967460, 227.8920494084358950, 45.00000000000000000 ) ) ;
#12715=DIRECTION ( 'NONE',  ( -0.000000000000000000, -0.000000000000000000, -1.000000000000000000 ) ) ;
#12738=CARTESIAN_POINT ( 'NONE',  ( 154.8288972274760908, 217.3894761555990556, 45.00000000000000000 ) ) ;
#12746=CARTESIAN_POINT ( 'NONE',  ( 48.74042075079900371, -13.05995637893015449, 45.00000000000000000 ) ) ;
#12757=AXIS2_PLACEMENT_3D ( 'NONE', #25168, #12259, #3326 ) ;
#12784=EDGE_LOOP ( 'NONE', ( #1028, #12809, #5058, #22014 ) ) ;
#12809=ORIENTED_EDGE ( 'NONE', *, *, #10080, .F. ) ;
#12835=DIRECTION ( 'NONE',  ( -0.8379557447115539848, -0.5457381880580697286, 0.000000000000000000 ) ) ;
#12837=LINE ( 'NONE', #10954, #10083 ) ;
#12857=EDGE_CURVE ( 'NONE', #10473, #25781, #17344, .T. ) ;
#12875=CARTESIAN_POINT ( 'NONE',  ( 114.5814157129579058, 230.6339745962151540, 45.00000000000000000 ) ) ;
#12891=ORIENTED_EDGE ( 'NONE', *, *, #26834, .T. ) ;
#12897=EDGE_CURVE ( 'NONE', #9201, #22969, #7292, .T. ) ;
#12907=PLANE ( 'NONE',  #11554 ) ;
#12921=AXIS2_PLACEMENT_3D ( 'NONE', #1650, #16751, #12592 ) ;
#12929=CARTESIAN_POINT ( 'NONE',  ( 134.6436608991879496, 206.7391133850113079, -45.00000000000000000 ) ) ;
#12932=DIRECTION ( 'NONE',  ( 0.8660254037844324904, -0.5000000000000105471, 0.000000000000000000 ) ) ;
#12935=CARTESIAN_POINT ( 'NONE',  ( 153.4775906502255509, 227.6536686473015436, -45.00000000000000000 ) ) ;
#12950=ORIENTED_EDGE ( 'NONE', *, *, #7155, .T. ) ;
#12951=VERTEX_POINT ( 'NONE', #13475 ) ;
#12955=ORIENTED_EDGE ( 'NONE', *, *, #22916, .F. ) ;
#12960=DIRECTION ( 'NONE',  ( -1.000000000000000000, 0.000000000000000000, 0.000000000000000000 ) ) ;
#12972=EDGE_CURVE ( 'NONE', #9172, #9499, #6852, .T. ) ;
#12980=CARTESIAN_POINT ( 'NONE',  ( 147.1752285801741493, 235.8670668058244644, -45.00000000000000000 ) ) ;
#12988=ORIENTED_EDGE ( 'NONE', *, *, #12857, .T. ) ;
#12990=VECTOR ( 'NONE', #27361, 1000.000000000000000 ) ;
#12998=EDGE_CURVE ( 'NONE', #12262, #25868, #2823, .T. ) ;
#13001=LINE ( 'NONE', #15571, #14391 ) ;
#13008=DIRECTION ( 'NONE',  ( 0.9659258262890670910, 0.2588190451025251804, 0.000000000000000000 ) ) ;
#13009=DIRECTION ( 'NONE',  ( 0.7440215159219069063, 0.6681556583950086781, 0.000000000000000000 ) ) ;
#13016=VERTEX_POINT ( 'NONE', #24954 ) ;
#13023=CARTESIAN_POINT ( 'NONE',  ( -50.01279441628821587, 86.62470095750859400, -45.00000000000000000 ) ) ;
#13029=VECTOR ( 'NONE', #20858, 999.9999999999998863 ) ;
#13035=ORIENTED_EDGE ( 'NONE', *, *, #26114, .F. ) ;
#13037=ADVANCED_FACE ( 'NONE', ( #11172 ), #19927, .F. ) ;
#13062=ORIENTED_EDGE ( 'NONE', *, *, #2401, .F. ) ;
#13063=EDGE_CURVE ( 'NONE', #4583, #28122, #19045, .T. ) ;
#13064=EDGE_CURVE ( 'NONE', #21431, #10405, #3242, .T. ) ;
#13066=ORIENTED_EDGE ( 'NONE', *, *, #9378, .F. ) ;
#13079=CARTESIAN_POINT ( 'NONE',  ( 128.0812361363530272, 198.0425250404537394, 45.00000000000000000 ) ) ;
#13098=EDGE_LOOP ( 'NONE', ( #7268, #20772, #24016, #12891 ) ) ;
#13103=DIRECTION ( 'NONE',  ( -1.000000000000000000, 0.000000000000000000, 0.000000000000000000 ) ) ;
#13104=EDGE_LOOP ( 'NONE', ( #10195, #7757, #6501, #4021 ) ) ;
#13118=ORIENTED_EDGE ( 'NONE', *, *, #26899, .T. ) ;
#13121=DIRECTION ( 'NONE',  ( -0.9784193629480845145, -0.2066290158914390329, 0.000000000000000000 ) ) ;
#13131=( NAMED_UNIT ( * ) SI_UNIT ( $, .STERADIAN. ) SOLID_ANGLE_UNIT ( ) );
#13137=EDGE_CURVE ( 'NONE', #8240, #9208, #14054, .T. ) ;
#13144=ORIENTED_EDGE ( 'NONE', *, *, #8181, .F. ) ;
#13147=DIRECTION ( 'NONE',  ( -0.7440215159218921404, 0.6681556583950252204, 0.000000000000000000 ) ) ;
#13151=CARTESIAN_POINT ( 'NONE',  ( 119.1329331941752230, 232.1752285801739220, 45.00000000000000000 ) ) ;
#13167=VECTOR ( 'NONE', #12715, 1000.000000000000000 ) ;
#13184=LINE ( 'NONE', #13322, #16528 ) ;
#13240=VECTOR ( 'NONE', #13576, 999.9999999999998863 ) ;
#13241=VERTEX_POINT ( 'NONE', #26069 ) ;
#13260=VERTEX_POINT ( 'NONE', #21909 ) ;
#13264=CARTESIAN_POINT ( 'NONE',  ( 203.1730087600953993, 54.44004362106413453, 45.00000000000000000 ) ) ;
#13280=DIRECTION ( 'NONE',  ( 0.6681556583950252204, 0.7440215159218921404, -0.000000000000000000 ) ) ;
#13282=DIRECTION ( 'NONE',  ( 0.9506505318133474658, -0.3102637045530776683, 0.000000000000000000 ) ) ;
#13284=DIRECTION ( 'NONE',  ( -0.000000000000000000, 0.000000000000000000, 1.000000000000000000 ) ) ;
#13285=EDGE_CURVE ( 'NONE', #15999, #15612, #11723, .T. ) ;
#13293=CARTESIAN_POINT ( 'NONE',  ( 154.4185842870419663, 232.3660254037841639, 45.00000000000000000 ) ) ;
#13309=ORIENTED_EDGE ( 'NONE', *, *, #27725, .F. ) ;
#13321=EDGE_CURVE ( 'NONE', #10473, #7097, #8979, .T. ) ;
#13322=CARTESIAN_POINT ( 'NONE',  ( 158.7404207507997853, 42.53436754635193040, -45.00000000000000000 ) ) ;
#13330=CARTESIAN_POINT ( 'NONE',  ( 197.6424708188942816, 64.50455043276784295, 45.00000000000000000 ) ) ;
#13343=ORIENTED_EDGE ( 'NONE', *, *, #13064, .F. ) ;
#13352=FACE_OUTER_BOUND ( 'NONE', #24417, .T. ) ;
#13361=FACE_OUTER_BOUND ( 'NONE', #3523, .T. ) ;
#13396=CARTESIAN_POINT ( 'NONE',  ( 146.9844428835009467, 225.6878133005969858, 45.00000000000000000 ) ) ;
#13405=EDGE_CURVE ( 'NONE', #8289, #5518, #25193, .T. ) ;
#13408=DIRECTION ( 'NONE',  ( -0.000000000000000000, -0.000000000000000000, -1.000000000000000000 ) ) ;
#13410=ORIENTED_EDGE ( 'NONE', *, *, #21318, .F. ) ;
#13431=PLANE ( 'NONE',  #6819 ) ;
#13435=VECTOR ( 'NONE', #16726, 1000.000000000000000 ) ;
#13437=FACE_OUTER_BOUND ( 'NONE', #26973, .T. ) ;
#13448=AXIS2_PLACEMENT_3D ( 'NONE', #24471, #7089, #22170 ) ;
#13455=ORIENTED_EDGE ( 'NONE', *, *, #2679, .T. ) ;
#13475=CARTESIAN_POINT ( 'NONE',  ( 124.3660254037845192, 199.5814157129575506, -45.00000000000000000 ) ) ;
#13479=VERTEX_POINT ( 'NONE', #14153 ) ;
#13483=ORIENTED_EDGE ( 'NONE', *, *, #900, .F. ) ;
#13486=EDGE_CURVE ( 'NONE', #999, #16719, #14026, .T. ) ;
#13493=LINE ( 'NONE', #20082, #12065 ) ;
#13531=CARTESIAN_POINT ( 'NONE',  ( 145.6339745962154097, 240.4185842870418242, -45.00000000000000000 ) ) ;
#13544=ORIENTED_EDGE ( 'NONE', *, *, #14366, .F. ) ;
#13549=ORIENTED_EDGE ( 'NONE', *, *, #6690, .F. ) ;
#13556=ORIENTED_EDGE ( 'NONE', *, *, #3339, .F. ) ;
#13576=DIRECTION ( 'NONE',  ( -0.3102637045530707294, -0.9506505318133497973, 0.000000000000000000 ) ) ;
#13578=CARTESIAN_POINT ( 'NONE',  ( 122.6339745962156229, 200.5814157129576074, -45.00000000000000000 ) ) ;
#13579=CARTESIAN_POINT ( 'NONE',  ( 154.8288972274760908, 217.3894761555990556, -45.00000000000000000 ) ) ;
#13581=ORIENTED_EDGE ( 'NONE', *, *, #2890, .F. ) ;
#13600=DIRECTION ( 'NONE',  ( -1.387778780781444256E-14, -1.000000000000000000, 0.000000000000000000 ) ) ;
#13607=CARTESIAN_POINT ( 'NONE',  ( 95.82124051657368113, -20.23615780638419182, -45.00000000000000000 ) ) ;
#13641=DIRECTION ( 'NONE',  ( -0.3102637045530823867, -0.9506505318133460225, 0.000000000000000000 ) ) ;
#13655=FACE_OUTER_BOUND ( 'NONE', #23011, .T. ) ;
#13669=EDGE_CURVE ( 'NONE', #3329, #15219, #617, .T. ) ;
#13674=EDGE_CURVE ( 'NONE', #23094, #13728, #15994, .T. ) ;
#13676=ORIENTED_EDGE ( 'NONE', *, *, #8794, .T. ) ;
#13677=LINE ( 'NONE', #9166, #3157 ) ;
#13717=CARTESIAN_POINT ( 'NONE',  ( 154.8288972274760908, 222.6105238444010297, -45.00000000000000000 ) ) ;
#13721=CARTESIAN_POINT ( 'NONE',  ( 111.9999999999999574, 220.9999999999996874, 45.00000000000000000 ) ) ;
#13727=LINE ( 'NONE', #14016, #9141 ) ;
#13728=VERTEX_POINT ( 'NONE', #20703 ) ;
#13746=ORIENTED_EDGE ( 'NONE', *, *, #570, .T. ) ;
#13756=DIRECTION ( 'NONE',  ( 0.7440215159219103480, 0.6681556583950049033, -0.000000000000000000 ) ) ;
#13764=CARTESIAN_POINT ( 'NONE',  ( 155.4185842870420799, 209.3660254037844481, 45.00000000000000000 ) ) ;
#13767=ADVANCED_FACE ( 'NONE', ( #2902 ), #14393, .F. ) ;
#13769=DIRECTION ( 'NONE',  ( -0.3102637045530683979, 0.9506505318133506854, 0.000000000000000000 ) ) ;
#13779=EDGE_CURVE ( 'NONE', #9244, #11167, #5336, .T. ) ;
#13784=VECTOR ( 'NONE', #2925, 1000.000000000000000 ) ;
#13802=LINE ( 'NONE', #9620, #25199 ) ;
#13822=ORIENTED_EDGE ( 'NONE', *, *, #17613, .T. ) ;
#13833=DIRECTION ( 'NONE',  ( -0.6681556583950049033, 0.7440215159219103480, 0.000000000000000000 ) ) ;
#13834=ORIENTED_EDGE ( 'NONE', *, *, #6764, .F. ) ;
#13837=ADVANCED_FACE ( 'NONE', ( #23148 ), #3311, .F. ) ;
#13840=VERTEX_POINT ( 'NONE', #20424 ) ;
#13876=LINE ( 'NONE', #17880, #4131 ) ;
#13919=CARTESIAN_POINT ( 'NONE',  ( 115.1711027725237528, 222.6105238444006886, 45.00000000000000000 ) ) ;
#13926=ORIENTED_EDGE ( 'NONE', *, *, #4655, .F. ) ;
#13930=CARTESIAN_POINT ( 'NONE',  ( 67.86343429515802939, -22.14858123305036486, 45.00000000000000000 ) ) ;
#13945=DIRECTION ( 'NONE',  ( -0.8916010070293515222, 0.4528218681382848443, 0.000000000000000000 ) ) ;
#13955=DIRECTION ( 'NONE',  ( -0.9985600561963485777, -0.05364526231779759985, 0.000000000000000000 ) ) ;
#13969=DIRECTION ( 'NONE',  ( 0.9784193629480785193, -0.2066290158914672881, 0.000000000000000000 ) ) ;
#13979=AXIS2_PLACEMENT_3D ( 'NONE', #23737, #12835, #1892 ) ;
#13983=CARTESIAN_POINT ( 'NONE',  ( 142.6536686473015152, 238.4775906502254941, -45.00000000000000000 ) ) ;
#13989=EDGE_LOOP ( 'NONE', ( #14821, #9776, #13834, #2654 ) ) ;
#14016=CARTESIAN_POINT ( 'NONE',  ( 197.6424708188942816, 64.50455043276784295, -45.00000000000000000 ) ) ;
#14026=CIRCLE ( 'NONE', #10781, 10.00000000000000888 ) ;
#14034=AXIS2_PLACEMENT_3D ( 'NONE', #10095, #15228, #5494 ) ;
#14035=VERTEX_POINT ( 'NONE', #7040 ) ;
#14048=CARTESIAN_POINT ( 'NONE',  ( 150.5563491861038870, 236.9705627484768797, 45.00000000000000000 ) ) ;
#14054=LINE ( 'NONE', #1238, #3405 ) ;
#14060=ORIENTED_EDGE ( 'NONE', *, *, #14287, .T. ) ;
#14065=ORIENTED_EDGE ( 'NONE', *, *, #28147, .T. ) ;
#14096=EDGE_CURVE ( 'NONE', #14325, #28186, #8682, .T. ) ;
#14105=CLOSED_SHELL ( 'NONE', ( #24733, #24368, #15472, #5519, #11628, #16035, #25271, #9322, #21577, #19402, #23662, #2507, #2166, #3759, #7594, #6782, #28238, #19055, #8248, #26199, #18302, #20481, #1083, #13037, #8532, #4475, #14113, #19363, #20226, #16117, #19569, #3512, #18600, #24825, #1844, #4686, #315, #5742, #3376, #2232, #1341, #343, #23568, #5838, #27586, #27731, #12367, #26459, #6452, #2075, #6617, #14823, #24245, #4669, #11849, #22203, #2732, #23695, #24865, #10603, #9650, #20395, #11294, #11903, #11707, #13767, #20183, #12441, #13837, #11245, #19049, #22356, #14230, #25555, #21271, #8585 ) ) ;
#14112=EDGE_CURVE ( 'NONE', #13260, #5560, #6378, .T. ) ;
#14113=ADVANCED_FACE ( 'NONE', ( #17576 ), #19313, .F. ) ;
#14151=DIRECTION ( 'NONE',  ( -0.8379557447115514313, 0.5457381880580733924, 0.000000000000000000 ) ) ;
#14152=CARTESIAN_POINT ( 'NONE',  ( -66.57029700917655646, 102.2156118568357783, 45.00000000000000000 ) ) ;
#14153=CARTESIAN_POINT ( 'NONE',  ( 115.1711027725237955, 217.3894761555985156, 45.00000000000000000 ) ) ;
#14203=EDGE_CURVE ( 'NONE', #9208, #4554, #10981, .T. ) ;
#14223=VERTEX_POINT ( 'NONE', #3613 ) ;
#14224=ORIENTED_EDGE ( 'NONE', *, *, #14112, .T. ) ;
#14230=ADVANCED_FACE ( 'NONE', ( #16428 ), #22886, .F. ) ;
#14233=ORIENTED_EDGE ( 'NONE', *, *, #3460, .T. ) ;
#14235=DIRECTION ( 'NONE',  ( -0.05364526231778202897, 0.9985600561963492439, 0.000000000000000000 ) ) ;
#14238=EDGE_CURVE ( 'NONE', #11167, #27470, #10239, .T. ) ;
#14249=CARTESIAN_POINT ( 'NONE',  ( 127.3463313526980727, 238.4775906502252667, 45.00000000000000000 ) ) ;
#14254=DIRECTION ( 'NONE',  ( -0.9985600561963489108, 0.05364526231778980747, 0.000000000000000000 ) ) ;
#14258=VECTOR ( 'NONE', #8611, 1000.000000000000000 ) ;
#14269=ORIENTED_EDGE ( 'NONE', *, *, #10835, .F. ) ;
#14287=EDGE_CURVE ( 'NONE', #5668, #3350, #21145, .T. ) ;
#14292=DIRECTION ( 'NONE',  ( -0.8379557447115656421, -0.5457381880580516320, 0.000000000000000000 ) ) ;
#14312=LINE ( 'NONE', #5111, #12990 ) ;
#14322=DIRECTION ( 'NONE',  ( -0.05364526231779676024, -0.9985600561963485777, 0.000000000000000000 ) ) ;
#14324=CARTESIAN_POINT ( 'NONE',  ( 0.000000000000000000, 0.000000000000000000, -45.00000000000000000 ) ) ;
#14325=VERTEX_POINT ( 'NONE', #12267 ) ;
#14366=EDGE_CURVE ( 'NONE', #11107, #23094, #15659, .T. ) ;
#14368=ORIENTED_EDGE ( 'NONE', *, *, #6864, .T. ) ;
#14375=VECTOR ( 'NONE', #16306, 999.9999999999998863 ) ;
#14376=CARTESIAN_POINT ( 'NONE',  ( 135.9999999999998295, 242.9999999999997158, -45.00000000000000000 ) ) ;
#14391=VECTOR ( 'NONE', #26326, 1000.000000000000114 ) ;
#14393=PLANE ( 'NONE',  #26857 ) ;
#14411=DIRECTION ( 'NONE',  ( -0.000000000000000000, -0.000000000000000000, -1.000000000000000000 ) ) ;
#14436=AXIS2_PLACEMENT_3D ( 'NONE', #10375, #6059, #23590 ) ;
#14482=LINE ( 'NONE', #18780, #7700 ) ;
#14490=AXIS2_PLACEMENT_3D ( 'NONE', #8680, #13280, #13147 ) ;
#14498=DIRECTION ( 'NONE',  ( 0.3102637045530823312, 0.9506505318133460225, 0.000000000000000000 ) ) ;
#14526=CARTESIAN_POINT ( 'NONE',  ( 161.2365440327092472, 161.2365440327092472, 45.00000000000000000 ) ) ;
#14532=ORIENTED_EDGE ( 'NONE', *, *, #21820, .F. ) ;
#14543=PLANE ( 'NONE',  #12757 ) ;
#14550=EDGE_CURVE ( 'NONE', #11738, #6712, #27262, .T. ) ;
#14562=DIRECTION ( 'NONE',  ( 0.4999999999999985012, 0.8660254037844394848, 0.000000000000000000 ) ) ;
#14577=ORIENTED_EDGE ( 'NONE', *, *, #13285, .T. ) ;
#14598=PLANE ( 'NONE',  #25613 ) ;
#14605=DIRECTION ( 'NONE',  ( -0.000000000000000000, -0.000000000000000000, -1.000000000000000000 ) ) ;
#14625=PRODUCT_DEFINITION_SHAPE ( 'NONE', 'NONE',  #6305 ) ;
#14632=CARTESIAN_POINT ( 'NONE',  ( 115.5814157129578916, 232.3660254037840502, 45.00000000000000000 ) ) ;
#14636=VERTEX_POINT ( 'NONE', #10452 ) ;
#14643=ORIENTED_EDGE ( 'NONE', *, *, #8651, .T. ) ;
#14658=CARTESIAN_POINT ( 'NONE',  ( -0.000000000000000000, 196.9999999999997442, -45.00000000000000000 ) ) ;
#14659=AXIS2_PLACEMENT_3D ( 'NONE', #18099, #20388, #9485 ) ;
#14661=LINE ( 'NONE', #12379, #4065 ) ;
#14689=FACE_OUTER_BOUND ( 'NONE', #21695, .T. ) ;
#14695=ORIENTED_EDGE ( 'NONE', *, *, #14838, .F. ) ;
#14696=VECTOR ( 'NONE', #15340, 1000.000000000000000 ) ;
#14698=CARTESIAN_POINT ( 'NONE',  ( -41.54405845664282282, 46.26118624020713099, 45.00000000000000000 ) ) ;
#14718=LINE ( 'NONE', #23469, #3015 ) ;
#14719=VERTEX_POINT ( 'NONE', #21931 ) ;
#14720=ORIENTED_EDGE ( 'NONE', *, *, #21599, .T. ) ;
#14723=VECTOR ( 'NONE', #25498, 1000.000000000000000 ) ;
#14740=PLANE ( 'NONE',  #9117 ) ;
#14778=LINE ( 'NONE', #25680, #16496 ) ;
#14790=STYLED_ITEM('',(#28427),#8903);
#14813=DIRECTION ( 'NONE',  ( 0.7071067811865474617, -0.7071067811865474617, 0.000000000000000000 ) ) ;
#14821=ORIENTED_EDGE ( 'NONE', *, *, #3005, .T. ) ;
#14823=ADVANCED_FACE ( 'NONE', ( #950 ), #20768, .F. ) ;
#14838=EDGE_CURVE ( 'NONE', #23257, #19128, #9719, .T. ) ;
#14844=CARTESIAN_POINT ( 'NONE',  ( 111.9999999999999289, 218.9999999999996874, 45.00000000000000000 ) ) ;
#14847=VECTOR ( 'NONE', #14151, 1000.000000000000114 ) ;
#14852=VECTOR ( 'NONE', #25505, 1000.000000000000000 ) ;
#14860=DIRECTION ( 'NONE',  ( 1.000000000000000000, 0.000000000000000000, 0.000000000000000000 ) ) ;
#14878=EDGE_CURVE ( 'NONE', #12331, #9062, #16197, .T. ) ;
#14890=DIRECTION ( 'NONE',  ( -0.000000000000000000, -0.000000000000000000, -1.000000000000000000 ) ) ;
#14894=DIRECTION ( 'NONE',  ( 1.000000000000000000, 0.000000000000000000, 0.000000000000000000 ) ) ;
#14901=ORIENTED_EDGE ( 'NONE', *, *, #6756, .F. ) ;
#14917=DIRECTION ( 'NONE',  ( -0.8660254037844326014, 0.5000000000000106581, 0.000000000000000000 ) ) ;
#14923=DIRECTION ( 'NONE',  ( -0.000000000000000000, -0.000000000000000000, -1.000000000000000000 ) ) ;
#14925=ORIENTED_EDGE ( 'NONE', *, *, #3309, .T. ) ;
#14926=VERTEX_POINT ( 'NONE', #27092 ) ;
#14937=CARTESIAN_POINT ( 'NONE',  ( 147.1752285801744904, 204.1329331941753082, 45.00000000000000000 ) ) ;
#14940=VECTOR ( 'NONE', #13008, 1000.000000000000000 ) ;
#14944=DIRECTION ( 'NONE',  ( -0.000000000000000000, -0.000000000000000000, -1.000000000000000000 ) ) ;
#14947=VECTOR ( 'NONE', #6663, 1000.000000000000000 ) ;
#14991=ORIENTED_EDGE ( 'NONE', *, *, #5580, .F. ) ;
#14992=CARTESIAN_POINT ( 'NONE',  ( 122.8247714198253959, 235.8670668058242939, 45.00000000000000000 ) ) ;
#15006=DIRECTION ( 'NONE',  ( 0.8916010070293437506, -0.4528218681383003874, 0.000000000000000000 ) ) ;
#15009=VERTEX_POINT ( 'NONE', #27920 ) ;
#15010=ORIENTED_EDGE ( 'NONE', *, *, #1754, .T. ) ;
#15015=LINE ( 'NONE', #21183, #27098 ) ;
#15056=DIRECTION ( 'NONE',  ( 0.7071067811865613395, 0.7071067811865336949, 0.000000000000000000 ) ) ;
#15080=VECTOR ( 'NONE', #19640, 1000.000000000000000 ) ;
#15081=AXIS2_PLACEMENT_3D ( 'NONE', #3264, #1121, #18786 ) ;
#15082=CARTESIAN_POINT ( 'NONE',  ( 93.17300876009500143, -24.96563245364655259, -45.00000000000000000 ) ) ;
#15083=CARTESIAN_POINT ( 'NONE',  ( -58.76345596729049703, 58.76345596729049703, 45.00000000000000000 ) ) ;
#15086=CARTESIAN_POINT ( 'NONE',  ( 127.3463313526980727, 238.4775906502252667, -45.00000000000000000 ) ) ;
#15104=AXIS2_PLACEMENT_3D ( 'NONE', #20859, #11974, #18843 ) ;
#15107=CARTESIAN_POINT ( 'NONE',  ( 157.9999999999998579, 0.000000000000000000, 45.00000000000000000 ) ) ;
#15141=DIRECTION ( 'NONE',  ( -0.9659258262890662028, 0.2588190451025286221, 0.000000000000000000 ) ) ;
#15143=VERTEX_POINT ( 'NONE', #22038 ) ;
#15149=EDGE_CURVE ( 'NONE', #8625, #1736, #2068, .T. ) ;
#15150=EDGE_LOOP ( 'NONE', ( #27240, #4956, #1355, #15394 ) ) ;
#15169=CARTESIAN_POINT ( 'NONE',  ( 112.5248869502488986, 215.0130877889307044, 45.00000000000000000 ) ) ;
#15178=CARTESIAN_POINT ( 'NONE',  ( 150.8670668058245212, 232.1752285801742630, 45.00000000000000000 ) ) ;
#15181=ORIENTED_EDGE ( 'NONE', *, *, #27696, .F. ) ;
#15219=VERTEX_POINT ( 'NONE', #20593 ) ;
#15228=DIRECTION ( 'NONE',  ( -0.5457381880580680633, 0.8379557447115549840, 0.000000000000000000 ) ) ;
#15234=EDGE_CURVE ( 'NONE', #7395, #11330, #7099, .T. ) ;
#15265=EDGE_CURVE ( 'NONE', #1736, #6015, #9255, .T. ) ;
#15274=FACE_OUTER_BOUND ( 'NONE', #7301, .T. ) ;
#15304=DIRECTION ( 'NONE',  ( 0.8379557447115657531, 0.5457381880580516320, 0.000000000000000000 ) ) ;
#15309=EDGE_CURVE ( 'NONE', #11692, #21431, #24626, .T. ) ;
#15313=ORIENTED_EDGE ( 'NONE', *, *, #12617, .T. ) ;
#15326=CARTESIAN_POINT ( 'NONE',  ( 118.0294372515226939, 235.5563491861037164, 45.00000000000000000 ) ) ;
#15328=VECTOR ( 'NONE', #19176, 1000.000000000000000 ) ;
#15337=EDGE_CURVE ( 'NONE', #962, #2873, #642, .T. ) ;
#15340=DIRECTION ( 'NONE',  ( -0.000000000000000000, -0.000000000000000000, -1.000000000000000000 ) ) ;
#15363=EDGE_LOOP ( 'NONE', ( #8280, #22951, #9848, #8567 ) ) ;
#15386=VECTOR ( 'NONE', #18867, 1000.000000000000000 ) ;
#15394=ORIENTED_EDGE ( 'NONE', *, *, #16814, .T. ) ;
#15402=LINE ( 'NONE', #26576, #5453 ) ;
#15405=VECTOR ( 'NONE', #11098, 999.9999999999998863 ) ;
#15437=ORIENTED_EDGE ( 'NONE', *, *, #6375, .F. ) ;
#15446=CARTESIAN_POINT ( 'NONE',  ( 155.4185842870420799, 209.3660254037844481, 45.00000000000000000 ) ) ;
#15457=DIRECTION ( 'NONE',  ( -0.5457381880580697286, 0.8379557447115539848, 0.000000000000000000 ) ) ;
#15472=ADVANCED_FACE ( 'NONE', ( #16436 ), #23032, .F. ) ;
#15478=DIRECTION ( 'NONE',  ( 0.6681556583950127859, 0.7440215159219033536, 0.000000000000000000 ) ) ;
#15502=ORIENTED_EDGE ( 'NONE', *, *, #6864, .F. ) ;
#15509=CARTESIAN_POINT ( 'NONE',  ( 73.69623568533953062, -15.56365422765611051, 45.00000000000000000 ) ) ;
#15563=CARTESIAN_POINT ( 'NONE',  ( 157.9999999999998579, 219.0000000000000284, 45.00000000000000000 ) ) ;
#15571=CARTESIAN_POINT ( 'NONE',  ( 3.660298066448477439, -2.383854334960948229, 45.00000000000000000 ) ) ;
#15572=ORIENTED_EDGE ( 'NONE', *, *, #17811, .T. ) ;
#15575=LINE ( 'NONE', #6376, #14940 ) ;
#15577=CARTESIAN_POINT ( 'NONE',  ( 81.39309752945497678, 249.3891174404998594, 45.00000000000000000 ) ) ;
#15578=DIRECTION ( 'NONE',  ( 0.8916010070293515222, 0.4528218681382848443, 0.000000000000000000 ) ) ;
#15580=LINE ( 'NONE', #17866, #9154 ) ;
#15588=DIRECTION ( 'NONE',  ( -0.000000000000000000, -0.000000000000000000, -1.000000000000000000 ) ) ;
#15589=ORIENTED_EDGE ( 'NONE', *, *, #12617, .F. ) ;
#15593=AXIS2_PLACEMENT_3D ( 'NONE', #12456, #8416, #17174 ) ;
#15597=DIRECTION ( 'NONE',  ( 0.9784193629480814058, 0.2066290158914539099, -0.000000000000000000 ) ) ;
#15610=EDGE_LOOP ( 'NONE', ( #13822, #20326, #19264, #23036 ) ) ;
#15612=VERTEX_POINT ( 'NONE', #26023 ) ;
#15613=ORIENTED_EDGE ( 'NONE', *, *, #26021, .T. ) ;
#15622=DIRECTION ( 'NONE',  ( -0.9985600561963485777, 0.05364526231779760679, 0.000000000000000000 ) ) ;
#15638=VECTOR ( 'NONE', #24375, 1000.000000000000000 ) ;
#15643=ORIENTED_EDGE ( 'NONE', *, *, #3281, .T. ) ;
#15653=CARTESIAN_POINT ( 'NONE',  ( 134.0000000000000853, 196.9999999999997442, 45.00000000000000000 ) ) ;
#15658=FACE_OUTER_BOUND ( 'NONE', #15610, .T. ) ;
#15659=LINE ( 'NONE', #7005, #17702 ) ;
#15666=DIRECTION ( 'NONE',  ( -0.3102637045530588500, 0.9506505318133535720, 0.000000000000000000 ) ) ;
#15681=ORIENTED_EDGE ( 'NONE', *, *, #22756, .F. ) ;
#15709=LINE ( 'NONE', #2324, #6056 ) ;
#15747=CARTESIAN_POINT ( 'NONE',  ( 147.1752285801741493, 235.8670668058244644, 45.00000000000000000 ) ) ;
#15759=ORIENTED_EDGE ( 'NONE', *, *, #5831, .F. ) ;
#15761=VECTOR ( 'NONE', #15056, 1000.000000000000000 ) ;
#15776=EDGE_LOOP ( 'NONE', ( #9196, #4561, #16824, #13676 ) ) ;
#15784=AXIS2_PLACEMENT_3D ( 'NONE', #23494, #5965, #6388 ) ;
#15800=EDGE_CURVE ( 'NONE', #3728, #12262, #12378, .T. ) ;
#15809=PLANE ( 'NONE',  #16303 ) ;
#15818=ORIENTED_EDGE ( 'NONE', *, *, #25209, .T. ) ;
#15836=DIRECTION ( 'NONE',  ( 0.7071067811865475727, 0.7071067811865475727, -0.000000000000000000 ) ) ;
#15841=VECTOR ( 'NONE', #22938, 1000.000000000000114 ) ;
#15853=ORIENTED_EDGE ( 'NONE', *, *, #5786, .F. ) ;
#15881=CARTESIAN_POINT ( 'NONE',  ( 193.7634559672933676, 193.7634559672857790, 45.00000000000000000 ) ) ;
#15883=LINE ( 'NONE', #11425, #3369 ) ;
#15889=LINE ( 'NONE', #26480, #11170 ) ;
#15893=FACE_OUTER_BOUND ( 'NONE', #16938, .T. ) ;
#15895=CARTESIAN_POINT ( 'NONE',  ( 157.4751130497509450, 224.9869122110685566, 45.00000000000000000 ) ) ;
#15939=LINE ( 'NONE', #20655, #20636 ) ;
#15943=DIRECTION ( 'NONE',  ( -0.2066290158914389774, 0.9784193629480844034, 0.000000000000000000 ) ) ;
#15953=CARTESIAN_POINT ( 'NONE',  ( 25.90578987075423001, -14.95671475544977724, 45.00000000000000000 ) ) ;
#15959=VECTOR ( 'NONE', #16219, 1000.000000000000114 ) ;
#15994=LINE ( 'NONE', #22010, #15405 ) ;
#15995=ORIENTED_EDGE ( 'NONE', *, *, #8181, .T. ) ;
#15996=ORIENTED_EDGE ( 'NONE', *, *, #20287, .T. ) ;
#15999=VERTEX_POINT ( 'NONE', #7987 ) ;
#16026=DIRECTION ( 'NONE',  ( -0.000000000000000000, -0.000000000000000000, -1.000000000000000000 ) ) ;
#16035=ADVANCED_FACE ( 'NONE', ( #8127 ), #14598, .F. ) ;
#16048=VECTOR ( 'NONE', #26226, 1000.000000000000000 ) ;
#16058=DIRECTION ( 'NONE',  ( 0.9784193629480781862, -0.2066290158914688702, 0.000000000000000000 ) ) ;
#16060=DIRECTION ( 'NONE',  ( -1.000000000000000000, 0.000000000000000000, 0.000000000000000000 ) ) ;
#16078=DIRECTION ( 'NONE',  ( -0.7071067811865336949, 0.7071067811865613395, 0.000000000000000000 ) ) ;
#16083=EDGE_CURVE ( 'NONE', #5476, #13728, #16755, .T. ) ;
#16098=LINE ( 'NONE', #11355, #25356 ) ;
#16104=EDGE_CURVE ( 'NONE', #22985, #15009, #10712, .T. ) ;
#16117=ADVANCED_FACE ( 'NONE', ( #10566 ), #14740, .F. ) ;
#16140=CARTESIAN_POINT ( 'NONE',  ( 46.36636626309694975, -15.13258561588589757, 45.00000000000000000 ) ) ;
#16195=CARTESIAN_POINT ( 'NONE',  ( 121.6232796275294277, 239.4748271322486630, -45.00000000000000000 ) ) ;
#16197=LINE ( 'NONE', #16470, #27354 ) ;
#16201=CARTESIAN_POINT ( 'NONE',  ( 0.000000000000000000, 196.9999999999997442, 45.00000000000000000 ) ) ;
#16205=DIRECTION ( 'NONE',  ( 0.4999999999999881206, -0.8660254037844455910, 0.000000000000000000 ) ) ;
#16211=ORIENTED_EDGE ( 'NONE', *, *, #24532, .F. ) ;
#16214=VECTOR ( 'NONE', #9126, 1000.000000000000000 ) ;
#16218=ORIENTED_EDGE ( 'NONE', *, *, #13137, .F. ) ;
#16219=DIRECTION ( 'NONE',  ( 0.4528218681382910060, 0.8916010070293484135, 0.000000000000000000 ) ) ;
#16237=FACE_OUTER_BOUND ( 'NONE', #1279, .T. ) ;
#16283=LINE ( 'NONE', #20574, #11189 ) ;
#16286=CARTESIAN_POINT ( 'NONE',  ( -48.38593899427829115, 148.2549133597845241, -45.00000000000000000 ) ) ;
#16291=CARTESIAN_POINT ( 'NONE',  ( 176.5942101292460222, 101.9567147554491271, 45.00000000000000000 ) ) ;
#16297=EDGE_CURVE ( 'NONE', #11332, #19790, #7539, .T. ) ;
#16303=AXIS2_PLACEMENT_3D ( 'NONE', #6598, #17795, #9185 ) ;
#16306=DIRECTION ( 'NONE',  ( 0.5457381880580551847, -0.8379557447115634217, 0.000000000000000000 ) ) ;
#16321=LINE ( 'NONE', #26942, #1234 ) ;
#16337=LINE ( 'NONE', #25086, #22862 ) ;
#16342=EDGE_CURVE ( 'NONE', #194, #27280, #13727, .T. ) ;
#16344=DIRECTION ( 'NONE',  ( 0.8379557447115515423, -0.5457381880580733924, 0.000000000000000000 ) ) ;
#16345=AXIS2_PLACEMENT_3D ( 'NONE', #21962, #24403, #24262 ) ;
#16367=DIRECTION ( 'NONE',  ( 0.9659258262890670910, -0.2588190451025251804, 0.000000000000000000 ) ) ;
#16374=EDGE_CURVE ( 'NONE', #9499, #7395, #9689, .T. ) ;
#16376=DIRECTION ( 'NONE',  ( 0.000000000000000000, -1.000000000000000000, 0.000000000000000000 ) ) ;
#16416=ORIENTED_EDGE ( 'NONE', *, *, #7465, .T. ) ;
#16418=ORIENTED_EDGE ( 'NONE', *, *, #26021, .F. ) ;
#16428=FACE_OUTER_BOUND ( 'NONE', #10233, .T. ) ;
#16436=FACE_OUTER_BOUND ( 'NONE', #15150, .T. ) ;
#16438=DIRECTION ( 'NONE',  ( -0.7440215159218956931, 0.6681556583950213346, 0.000000000000000000 ) ) ;
#16440=ORIENTED_EDGE ( 'NONE', *, *, #11615, .F. ) ;
#16444=LINE ( 'NONE', #14152, #19267 ) ;
#16470=CARTESIAN_POINT ( 'NONE',  ( 134.1167547769962596, -7.205103435269982093, -45.00000000000000000 ) ) ;
#16490=VECTOR ( 'NONE', #9362, 1000.000000000000000 ) ;
#16496=VECTOR ( 'NONE', #14498, 1000.000000000000000 ) ;
#16502=PLANE ( 'NONE',  #15081 ) ;
#16517=CARTESIAN_POINT ( 'NONE',  ( 139.9869122110690114, 197.5248869502487139, 45.00000000000000000 ) ) ;
#16518=VERTEX_POINT ( 'NONE', #14992 ) ;
#16528=VECTOR ( 'NONE', #21927, 1000.000000000000114 ) ;
#16541=ORIENTED_EDGE ( 'NONE', *, *, #16850, .T. ) ;
#16544=CARTESIAN_POINT ( 'NONE',  ( -40.00387671809203738, 149.2965004116384762, 45.00000000000000000 ) ) ;
#16547=EDGE_CURVE ( 'NONE', #24909, #9062, #27612, .T. ) ;
#16551=CARTESIAN_POINT ( 'NONE',  ( 119.4436508138957720, 236.9705627484767376, 45.00000000000000000 ) ) ;
#16552=ORIENTED_EDGE ( 'NONE', *, *, #6073, .T. ) ;
#16559=PLANE ( 'NONE',  #27942 ) ;
#16561=CARTESIAN_POINT ( 'NONE',  ( 130.0130877889311591, 197.5248869502486571, -45.00000000000000000 ) ) ;
#16563=CARTESIAN_POINT ( 'NONE',  ( -55.40193461144291831, 169.7519813918499665, -45.00000000000000000 ) ) ;
#16580=CARTESIAN_POINT ( 'NONE',  ( 185.9255560592262100, 121.0883471088020116, -45.00000000000000000 ) ) ;
#16581=LINE ( 'NONE', #18590, #16992 ) ;
#16588=AXIS2_PLACEMENT_3D ( 'NONE', #19461, #19174, #8408 ) ;
#16595=CARTESIAN_POINT ( 'NONE',  ( 119.1329331941753225, 207.8247714198252254, 45.00000000000000000 ) ) ;
#16599=ORIENTED_EDGE ( 'NONE', *, *, #25383, .T. ) ;
#16611=DIRECTION ( 'NONE',  ( -0.000000000000000000, -0.000000000000000000, -1.000000000000000000 ) ) ;
#16612=CARTESIAN_POINT ( 'NONE',  ( 119.1329331941753225, 207.8247714198252254, 45.00000000000000000 ) ) ;
#16617=LINE ( 'NONE', #18621, #18361 ) ;
#16622=LINE ( 'NONE', #21062, #25360 ) ;
#16636=VECTOR ( 'NONE', #27545, 1000.000000000000000 ) ;
#16645=DIRECTION ( 'NONE',  ( 0.3102637045530753368, 0.9506505318133483540, -0.000000000000000000 ) ) ;
#16649=EDGE_CURVE ( 'NONE', #26105, #8289, #12837, .T. ) ;
#16651=CARTESIAN_POINT ( 'NONE',  ( 0.000000000000000000, 242.9999999999997158, 45.00000000000000000 ) ) ;
#16652=EDGE_LOOP ( 'NONE', ( #9455, #12357, #19361, #12950 ) ) ;
#16667=VECTOR ( 'NONE', #7398, 1000.000000000000114 ) ;
#16669=AXIS2_PLACEMENT_3D ( 'NONE', #13330, #22079, #22934 ) ;
#16674=LINE ( 'NONE', #14658, #2417 ) ;
#16717=VERTEX_POINT ( 'NONE', #13983 ) ;
#16719=VERTEX_POINT ( 'NONE', #18273 ) ;
#16722=DIRECTION ( 'NONE',  ( 0.9659258262890662028, -0.2588190451025286221, 0.000000000000000000 ) ) ;
#16726=DIRECTION ( 'NONE',  ( -0.000000000000000000, -0.000000000000000000, -1.000000000000000000 ) ) ;
#16751=DIRECTION ( 'NONE',  ( -0.6681556583950213346, -0.7440215159218956931, 0.000000000000000000 ) ) ;
#16753=LINE ( 'NONE', #1092, #14852 ) ;
#16755=LINE ( 'NONE', #19043, #1763 ) ;
#16762=CARTESIAN_POINT ( 'NONE',  ( 124.3660254037845192, 199.5814157129575506, 45.00000000000000000 ) ) ;
#16785=PLANE ( 'NONE',  #26728 ) ;
#16788=EDGE_CURVE ( 'NONE', #22236, #21431, #7069, .T. ) ;
#16814=EDGE_CURVE ( 'NONE', #7917, #3880, #4903, .T. ) ;
#16824=ORIENTED_EDGE ( 'NONE', *, *, #12670, .F. ) ;
#16831=ORIENTED_EDGE ( 'NONE', *, *, #14287, .F. ) ;
#16850=EDGE_CURVE ( 'NONE', #10085, #627, #1302, .T. ) ;
#16855=CARTESIAN_POINT ( 'NONE',  ( 147.3660254037842492, 239.4185842870417673, 45.00000000000000000 ) ) ;
#16859=DIRECTION ( 'NONE',  ( -0.2588190451025286221, -0.9659258262890662028, 0.000000000000000000 ) ) ;
#16861=ORIENTED_EDGE ( 'NONE', *, *, #3717, .T. ) ;
#16875=AXIS2_PLACEMENT_3D ( 'NONE', #5433, #23249, #25115 ) ;
#16887=CARTESIAN_POINT ( 'NONE',  ( 3.660298066448477439, -2.383854334960948229, 45.00000000000000000 ) ) ;
#16888=EDGE_CURVE ( 'NONE', #23507, #17680, #5891, .T. ) ;
#16896=ORIENTED_EDGE ( 'NONE', *, *, #24433, .F. ) ;
#16926=DIRECTION ( 'NONE',  ( 0.05364526231779759985, 0.9985600561963485777, 0.000000000000000000 ) ) ;
#16938=EDGE_LOOP ( 'NONE', ( #16541, #22777, #16831, #17703 ) ) ;
#16949=CARTESIAN_POINT ( 'NONE',  ( 157.9999999999998579, 219.0000000000000284, 45.00000000000000000 ) ) ;
#16965=CARTESIAN_POINT ( 'NONE',  ( 154.4185842870420799, 207.6339745962155803, 45.00000000000000000 ) ) ;
#16978=CARTESIAN_POINT ( 'NONE',  ( 46.36636626309694975, -15.13258561588589757, 45.00000000000000000 ) ) ;
#16989=DIRECTION ( 'NONE',  ( -0.000000000000000000, -0.000000000000000000, -1.000000000000000000 ) ) ;
#16992=VECTOR ( 'NONE', #5513, 1000.000000000000114 ) ;
#16998=ORIENTED_EDGE ( 'NONE', *, *, #13674, .F. ) ;
#16999=CARTESIAN_POINT ( 'NONE',  ( 132.3894761555988282, 239.8288972274758919, 45.00000000000000000 ) ) ;
#17020=VECTOR ( 'NONE', #5027, 1000.000000000000000 ) ;
#17050=VECTOR ( 'NONE', #475, 999.9999999999998863 ) ;
#17054=CARTESIAN_POINT ( 'NONE',  ( -66.57029700917655646, 102.2156118568357783, 45.00000000000000000 ) ) ;
#17057=LINE ( 'NONE', #25814, #5738 ) ;
#17082=LINE ( 'NONE', #12233, #24951 ) ;
#17087=AXIS2_PLACEMENT_3D ( 'NONE', #22401, #1126, #25538 ) ;
#17089=CARTESIAN_POINT ( 'NONE',  ( 141.9187638636471434, 198.0425250404537678, 45.00000000000000000 ) ) ;
#17091=( GEOMETRIC_REPRESENTATION_CONTEXT ( 3 ) GLOBAL_UNCERTAINTY_ASSIGNED_CONTEXT ( ( #2554 ) ) GLOBAL_UNIT_ASSIGNED_CONTEXT ( ( #11582, #11861, #4942 ) ) REPRESENTATION_CONTEXT ( 'NONE', 'WORKASPACE' ) );
#17105=EDGE_LOOP ( 'NONE', ( #8463, #18833, #17218, #3472 ) ) ;
#17112=VECTOR ( 'NONE', #22367, 999.9999999999998863 ) ;
#17129=CARTESIAN_POINT ( 'NONE',  ( 184.7759657584203694, 39.02219989801907474, 45.00000000000000000 ) ) ;
#17133=FACE_OUTER_BOUND ( 'NONE', #25543, .T. ) ;
#17139=DIRECTION ( 'NONE',  ( -0.000000000000000000, 0.000000000000000000, 1.000000000000000000 ) ) ;
#17161=ORIENTED_EDGE ( 'NONE', *, *, #2234, .T. ) ;
#17174=DIRECTION ( 'NONE',  ( -0.8660254037844394848, 0.4999999999999985012, 0.000000000000000000 ) ) ;
#17176=LINE ( 'NONE', #6680, #27141 ) ;
#17178=VECTOR ( 'NONE', #13833, 1000.000000000000114 ) ;
#17218=ORIENTED_EDGE ( 'NONE', *, *, #12897, .F. ) ;
#17241=ORIENTED_EDGE ( 'NONE', *, *, #12644, .F. ) ;
#17266=VECTOR ( 'NONE', #2203, 1000.000000000000227 ) ;
#17268=DIRECTION ( 'NONE',  ( 0.4999999999999985012, 0.8660254037844394848, 0.000000000000000000 ) ) ;
#17273=EDGE_CURVE ( 'NONE', #11167, #20475, #809, .T. ) ;
#17279=ORIENTED_EDGE ( 'NONE', *, *, #20956, .F. ) ;
#17284=EDGE_LOOP ( 'NONE', ( #25774, #27068, #23756, #21304 ) ) ;
#17291=PLANE ( 'NONE',  #14490 ) ;
#17300=FACE_OUTER_BOUND ( 'NONE', #8631, .T. ) ;
#17302=FACE_OUTER_BOUND ( 'NONE', #6676, .T. ) ;
#17310=LINE ( 'NONE', #26351, #25292 ) ;
#17317=ORIENTED_EDGE ( 'NONE', *, *, #9657, .F. ) ;
#17344=LINE ( 'NONE', #10605, #8011 ) ;
#17348=ORIENTED_EDGE ( 'NONE', *, *, #9378, .T. ) ;
#17372=LINE ( 'NONE', #18382, #21995 ) ;
#17399=ORIENTED_EDGE ( 'NONE', *, *, #22847, .F. ) ;
#17422=LINE ( 'NONE', #11103, #7447 ) ;
#17426=CARTESIAN_POINT ( 'NONE',  ( 12.78000883847031588, 237.8887863075477469, -45.00000000000000000 ) ) ;
#17442=CARTESIAN_POINT ( 'NONE',  ( 156.9574749595459764, 213.0812361363529988, -45.00000000000000000 ) ) ;
#17467=CARTESIAN_POINT ( 'NONE',  ( 52.57751368840760620, 248.9624084326366358, -45.00000000000000000 ) ) ;
#17532=AXIS2_PLACEMENT_3D ( 'NONE', #626, #25166, #20296 ) ;
#17536=ORIENTED_EDGE ( 'NONE', *, *, #4631, .F. ) ;
#17543=EDGE_CURVE ( 'NONE', #19790, #4525, #26652, .T. ) ;
#17548=FACE_OUTER_BOUND ( 'NONE', #5283, .T. ) ;
#17553=AXIS2_PLACEMENT_3D ( 'NONE', #9624, #17951, #15666 ) ;
#17554=EDGE_CURVE ( 'NONE', #5169, #14223, #2519, .T. ) ;
#17576=FACE_OUTER_BOUND ( 'NONE', #22020, .T. ) ;
#17578=LINE ( 'NONE', #11417, #27006 ) ;
#17595=ORIENTED_EDGE ( 'NONE', *, *, #9091, .F. ) ;
#17600=ORIENTED_EDGE ( 'NONE', *, *, #8134, .F. ) ;
#17613=EDGE_CURVE ( 'NONE', #9726, #10441, #13184, .T. ) ;
#17617=CARTESIAN_POINT ( 'NONE',  ( 116.5224093497741364, 227.6536686473013447, -45.00000000000000000 ) ) ;
#17628=CARTESIAN_POINT ( 'NONE',  ( 162.6509609271901411, 34.34969631929494938, 45.00000000000000000 ) ) ;
#17629=ORIENTED_EDGE ( 'NONE', *, *, #27755, .F. ) ;
#17649=LINE ( 'NONE', #22104, #1094 ) ;
#17674=ORIENTED_EDGE ( 'NONE', *, *, #8652, .F. ) ;
#17680=VERTEX_POINT ( 'NONE', #17617 ) ;
#17697=AXIS2_PLACEMENT_3D ( 'NONE', #7079, #11398, #18146 ) ;
#17702=VECTOR ( 'NONE', #4859, 1000.000000000000114 ) ;
#17703=ORIENTED_EDGE ( 'NONE', *, *, #6375, .T. ) ;
#17708=PLANE ( 'NONE',  #8580 ) ;
#17734=CARTESIAN_POINT ( 'NONE',  ( 162.6509609271901411, 34.34969631929494938, 45.00000000000000000 ) ) ;
#17747=EDGE_CURVE ( 'NONE', #15219, #11070, #18613, .T. ) ;
#17767=DIRECTION ( 'NONE',  ( 0.4528218681382754074, -0.8916010070293562961, 0.000000000000000000 ) ) ;
#17784=DIRECTION ( 'NONE',  ( -0.9506505318133460225, 0.3102637045530823867, 0.000000000000000000 ) ) ;
#17786=LINE ( 'NONE', #12929, #23101 ) ;
#17790=CARTESIAN_POINT ( 'NONE',  ( 157.4751130497509450, 224.9869122110685566, 45.00000000000000000 ) ) ;
#17795=DIRECTION ( 'NONE',  ( -0.7440215159219033536, 0.6681556583950127859, 0.000000000000000000 ) ) ;
#17811=EDGE_CURVE ( 'NONE', #10728, #2611, #15015, .T. ) ;
#17847=CARTESIAN_POINT ( 'NONE',  ( 130.0130877889311591, 197.5248869502486571, 45.00000000000000000 ) ) ;
#17850=EDGE_LOOP ( 'NONE', ( #20847, #17600, #22469, #23748 ) ) ;
#17866=CARTESIAN_POINT ( 'NONE',  ( -66.57029700917655646, 102.2156118568357783, -45.00000000000000000 ) ) ;
#17873=LINE ( 'NONE', #21401, #414 ) ;
#17880=CARTESIAN_POINT ( 'NONE',  ( -36.37721155344281243, 172.2515494757248291, 45.00000000000000000 ) ) ;
#17881=DIRECTION ( 'NONE',  ( 0.8660254037844394848, 0.4999999999999985012, 0.000000000000000000 ) ) ;
#17885=EDGE_CURVE ( 'NONE', #25868, #13016, #18890, .T. ) ;
#17931=ORIENTED_EDGE ( 'NONE', *, *, #21386, .T. ) ;
#17934=AXIS2_PLACEMENT_3D ( 'NONE', #20872, #18714, #12409 ) ;
#17951=DIRECTION ( 'NONE',  ( 0.9506505318133536830, 0.3102637045530589055, -0.000000000000000000 ) ) ;
#17956=CARTESIAN_POINT ( 'NONE',  ( 151.9705627484771355, 204.4436508138959141, 45.00000000000000000 ) ) ;
#17999=EDGE_LOOP ( 'NONE', ( #28087, #23048, #3786, #1704 ) ) ;
#18030=CARTESIAN_POINT ( 'NONE',  ( 204.8742559748123426, 133.4291290931197977, -45.00000000000000000 ) ) ;
#18040=ORIENTED_EDGE ( 'NONE', *, *, #27241, .T. ) ;
#18043=VECTOR ( 'NONE', #16026, 1000.000000000000000 ) ;
#18062=CARTESIAN_POINT ( 'NONE',  ( 52.57751368840760620, 248.9624084326366358, 45.00000000000000000 ) ) ;
#18063=ORIENTED_EDGE ( 'NONE', *, *, #27019, .T. ) ;
#18077=VERTEX_POINT ( 'NONE', #25181 ) ;
#18086=VECTOR ( 'NONE', #26443, 1000.000000000000000 ) ;
#18087=PRODUCT_DEFINITION_CONTEXT ( 'detailed design', #2117, 'design' ) ;
#18090=CARTESIAN_POINT ( 'NONE',  ( 114.5814157129579058, 230.6339745962151540, 45.00000000000000000 ) ) ;
#18099=CARTESIAN_POINT ( 'NONE',  ( -10.78991826960876033, 200.8449754580304898, 45.00000000000000000 ) ) ;
#18124=VECTOR ( 'NONE', #15457, 999.9999999999998863 ) ;
#18132=CARTESIAN_POINT ( 'NONE',  ( 158.7404207507997853, 42.53436754635193040, 45.00000000000000000 ) ) ;
#18133=DIRECTION ( 'NONE',  ( -0.000000000000000000, -0.000000000000000000, -1.000000000000000000 ) ) ;
#18137=DIRECTION ( 'NONE',  ( -0.2588190451024993122, 0.9659258262890740854, 0.000000000000000000 ) ) ;
#18146=DIRECTION ( 'NONE',  ( 0.4999999999999864553, -0.8660254037844463681, 0.000000000000000000 ) ) ;
#18161=VECTOR ( 'NONE', #26796, 1000.000000000000114 ) ;
#18165=ORIENTED_EDGE ( 'NONE', *, *, #11402, .T. ) ;
#18175=LINE ( 'NONE', #27205, #14847 ) ;
#18189=ORIENTED_EDGE ( 'NONE', *, *, #5786, .T. ) ;
#18192=ORIENTED_EDGE ( 'NONE', *, *, #27072, .T. ) ;
#18222=ORIENTED_EDGE ( 'NONE', *, *, #16649, .F. ) ;
#18241=PLANE ( 'NONE',  #20255 ) ;
#18256=ORIENTED_EDGE ( 'NONE', *, *, #16104, .F. ) ;
#18262=FACE_OUTER_BOUND ( 'NONE', #10128, .T. ) ;
#18268=EDGE_CURVE ( 'NONE', #1554, #5169, #10101, .T. ) ;
#18271=DIRECTION ( 'NONE',  ( 0.5457381880580551847, -0.8379557447115634217, 0.000000000000000000 ) ) ;
#18273=CARTESIAN_POINT ( 'NONE',  ( 124.9999999999998579, 220.0000000000000284, -45.00000000000000000 ) ) ;
#18278=DIRECTION ( 'NONE',  ( -0.9784193629480814058, -0.2066290158914539099, 0.000000000000000000 ) ) ;
#18294=ORIENTED_EDGE ( 'NONE', *, *, #10198, .F. ) ;
#18302=ADVANCED_FACE ( 'NONE', ( #19280 ), #28022, .F. ) ;
#18316=DIRECTION ( 'NONE',  ( 0.9784193629480814058, 0.2066290158914539099, 0.000000000000000000 ) ) ;
#18335=VECTOR ( 'NONE', #9377, 999.9999999999998863 ) ;
#18341=AXIS2_PLACEMENT_3D ( 'NONE', #290, #6737, #8760 ) ;
#18352=DIRECTION ( 'NONE',  ( -0.000000000000000000, -0.000000000000000000, -1.000000000000000000 ) ) ;
#18361=VECTOR ( 'NONE', #5547, 1000.000000000000000 ) ;
#18371=LINE ( 'NONE', #18090, #11618 ) ;
#18375=DIRECTION ( 'NONE',  ( -0.4528218681382848443, -0.8916010070293515222, 0.000000000000000000 ) ) ;
#18382=CARTESIAN_POINT ( 'NONE',  ( 69.99612328191057031, 261.2290884209365345, 45.00000000000000000 ) ) ;
#18417=ORIENTED_EDGE ( 'NONE', *, *, #7486, .T. ) ;
#18426=LINE ( 'NONE', #5206, #1478 ) ;
#18438=FACE_OUTER_BOUND ( 'NONE', #27271, .T. ) ;
#18460=ORIENTED_EDGE ( 'NONE', *, *, #12650, .T. ) ;
#18476=AXIS2_PLACEMENT_3D ( 'NONE', #22415, #4882, #24996 ) ;
#18483=CARTESIAN_POINT ( 'NONE',  ( 93.17300876009500143, -24.96563245364655259, 45.00000000000000000 ) ) ;
#18525=FACE_OUTER_BOUND ( 'NONE', #16652, .T. ) ;
#18535=CARTESIAN_POINT ( 'NONE',  ( 111.9999999999968878, -1.554312234475174324E-12, 45.00000000000000000 ) ) ;
#18577=CARTESIAN_POINT ( 'NONE',  ( 134.9999999999998579, 220.0000000000000284, 45.00000000000000000 ) ) ;
#18587=CARTESIAN_POINT ( 'NONE',  ( 73.69623568533953062, -15.56365422765611051, 45.00000000000000000 ) ) ;
#18590=CARTESIAN_POINT ( 'NONE',  ( 117.5127944162877753, 203.5381304684075019, 45.00000000000000000 ) ) ;
#18593=VECTOR ( 'NONE', #17881, 1000.000000000000114 ) ;
#18600=ADVANCED_FACE ( 'NONE', ( #19354 ), #12907, .F. ) ;
#18610=LINE ( 'NONE', #13607, #1148 ) ;
#18613=LINE ( 'NONE', #26811, #24813 ) ;
#18621=CARTESIAN_POINT ( 'NONE',  ( 139.9869122110687840, 242.4751130497508314, 45.00000000000000000 ) ) ;
#18625=FACE_OUTER_BOUND ( 'NONE', #5444, .T. ) ;
#18627=EDGE_LOOP ( 'NONE', ( #11007, #17317, #14901, #16599 ) ) ;
#18634=VERTEX_POINT ( 'NONE', #10746 ) ;
#18639=EDGE_LOOP ( 'NONE', ( #2976, #16418, #9591, #14368 ) ) ;
#18640=CARTESIAN_POINT ( 'NONE',  ( 193.7634559672933676, 193.7634559672857790, -45.00000000000000000 ) ) ;
#18641=DIRECTION ( 'NONE',  ( 0.6681556583950049033, -0.7440215159219103480, 0.000000000000000000 ) ) ;
#18677=DIRECTION ( 'NONE',  ( -0.000000000000000000, -0.000000000000000000, -1.000000000000000000 ) ) ;
#18693=EDGE_CURVE ( 'NONE', #4982, #22164, #27680, .T. ) ;
#18695=ORIENTED_EDGE ( 'NONE', *, *, #15265, .F. ) ;
#18714=DIRECTION ( 'NONE',  ( -0.7440215159219103480, -0.6681556583950049033, 0.000000000000000000 ) ) ;
#18721=FACE_OUTER_BOUND ( 'NONE', #17999, .T. ) ;
#18737=ORIENTED_EDGE ( 'NONE', *, *, #9301, .F. ) ;
#18765=CARTESIAN_POINT ( 'NONE',  ( 186.0596930950812293, 94.49506802741289846, -45.00000000000000000 ) ) ;
#18772=DIRECTION ( 'NONE',  ( -0.000000000000000000, -0.000000000000000000, -1.000000000000000000 ) ) ;
#18776=VECTOR ( 'NONE', #6413, 1000.000000000000000 ) ;
#18780=CARTESIAN_POINT ( 'NONE',  ( 175.6862808370088089, 157.7720269260891826, -45.00000000000000000 ) ) ;
#18785=DIRECTION ( 'NONE',  ( -0.9506505318133474658, 0.3102637045530776683, 0.000000000000000000 ) ) ;
#18786=DIRECTION ( 'NONE',  ( -0.5457381880580551847, 0.8379557447115634217, 0.000000000000000000 ) ) ;
#18792=CARTESIAN_POINT ( 'NONE',  ( 112.5248869502488986, 215.0130877889307044, 45.00000000000000000 ) ) ;
#18803=DIRECTION ( 'NONE',  ( 0.9985600561963485777, 0.05364526231779760679, 0.000000000000000000 ) ) ;
#18830=VERTEX_POINT ( 'NONE', #22220 ) ;
#18833=ORIENTED_EDGE ( 'NONE', *, *, #3639, .F. ) ;
#18843=DIRECTION ( 'NONE',  ( 0.5457381880580733924, 0.8379557447115515423, 0.000000000000000000 ) ) ;
#18864=EDGE_LOOP ( 'NONE', ( #26718, #3677, #14991, #5983 ) ) ;
#18867=DIRECTION ( 'NONE',  ( -0.7440215159218956931, 0.6681556583950213346, 0.000000000000000000 ) ) ;
#18870=LINE ( 'NONE', #7959, #13435 ) ;
#18874=CARTESIAN_POINT ( 'NONE',  ( 142.6536686473019699, 201.5224093497741649, 45.00000000000000000 ) ) ;
#18890=LINE ( 'NONE', #8261, #14723 ) ;
#18891=LINE ( 'NONE', #19736, #732 ) ;
#18912=SHAPE_REPRESENTATION ( 'Drive Gear', ( #10637 ), #19371 ) ;
#18945=LINE ( 'NONE', #10186, #7474 ) ;
#18948=VERTEX_POINT ( 'NONE', #7838 ) ;
#18957=EDGE_CURVE ( 'NONE', #23507, #23933, #7283, .T. ) ;
#18962=CARTESIAN_POINT ( 'NONE',  ( 8.415662294793918363, -4.274104551145060604, 45.00000000000000000 ) ) ;
#18967=LINE ( 'NONE', #3585, #21149 ) ;
#18991=CARTESIAN_POINT ( 'NONE',  ( -56.02075117275366978, 110.3042093914830559, 45.00000000000000000 ) ) ;
#18997=VECTOR ( 'NONE', #18271, 999.9999999999998863 ) ;
#19023=LINE ( 'NONE', #16595, #13167 ) ;
#19025=ORIENTED_EDGE ( 'NONE', *, *, #16104, .T. ) ;
#19039=CARTESIAN_POINT ( 'NONE',  ( 153.4775906502256930, 212.3463313526982859, 45.00000000000000000 ) ) ;
#19043=CARTESIAN_POINT ( 'NONE',  ( 154.4185842870419663, 232.3660254037841639, 45.00000000000000000 ) ) ;
#19045=LINE ( 'NONE', #25228, #20864 ) ;
#19049=ADVANCED_FACE ( 'NONE', ( #17300 ), #28063, .F. ) ;
#19054=VECTOR ( 'NONE', #19531, 999.9999999999998863 ) ;
#19055=ADVANCED_FACE ( 'NONE', ( #21332 ), #5819, .F. ) ;
#19079=ORIENTED_EDGE ( 'NONE', *, *, #7266, .F. ) ;
#19096=DIRECTION ( 'NONE',  ( -0.000000000000000000, 0.000000000000000000, 1.000000000000000000 ) ) ;
#19128=VERTEX_POINT ( 'NONE', #13578 ) ;
#19174=DIRECTION ( 'NONE',  ( -0.8916010070293595158, -0.4528218681382693567, 0.000000000000000000 ) ) ;
#19176=DIRECTION ( 'NONE',  ( -0.000000000000000000, -0.000000000000000000, -1.000000000000000000 ) ) ;
#19201=LINE ( 'NONE', #10872, #24906 ) ;
#19207=PLANE ( 'NONE',  #395 ) ;
#19228=VERTEX_POINT ( 'NONE', #17442 ) ;
#19264=ORIENTED_EDGE ( 'NONE', *, *, #19789, .F. ) ;
#19267=VECTOR ( 'NONE', #14292, 1000.000000000000114 ) ;
#19280=FACE_OUTER_BOUND ( 'NONE', #1418, .T. ) ;
#19293=ORIENTED_EDGE ( 'NONE', *, *, #14878, .F. ) ;
#19309=VECTOR ( 'NONE', #609, 1000.000000000000114 ) ;
#19312=CARTESIAN_POINT ( 'NONE',  ( 122.8247714198256944, 204.1329331941749672, -45.00000000000000000 ) ) ;
#19313=PLANE ( 'NONE',  #27762 ) ;
#19316=ORIENTED_EDGE ( 'NONE', *, *, #27628, .T. ) ;
#19322=DIRECTION ( 'NONE',  ( -0.5457381880580733924, -0.8379557447115515423, 0.000000000000000000 ) ) ;
#19354=FACE_OUTER_BOUND ( 'NONE', #1361, .T. ) ;
#19361=ORIENTED_EDGE ( 'NONE', *, *, #12521, .F. ) ;
#19363=ADVANCED_FACE ( 'NONE', ( #7536 ), #24773, .F. ) ;
#19369=ORIENTED_EDGE ( 'NONE', *, *, #13285, .F. ) ;
#19371=( GEOMETRIC_REPRESENTATION_CONTEXT ( 3 ) GLOBAL_UNCERTAINTY_ASSIGNED_CONTEXT ( ( #26402 ) ) GLOBAL_UNIT_ASSIGNED_CONTEXT ( ( #26034, #24037, #13131 ) ) REPRESENTATION_CONTEXT ( 'NONE', 'WORKASPACE' ) );
#19376=ORIENTED_EDGE ( 'NONE', *, *, #3300, .F. ) ;
#19377=LINE ( 'NONE', #26264, #22379 ) ;
#19387=CARTESIAN_POINT ( 'NONE',  ( 153.4775906502255509, 227.6536686473015436, 45.00000000000000000 ) ) ;
#19399=EDGE_CURVE ( 'NONE', #26105, #6540, #7392, .T. ) ;
#19402=ADVANCED_FACE ( 'NONE', ( #18721 ), #7100, .F. ) ;
#19438=ORIENTED_EDGE ( 'NONE', *, *, #12644, .T. ) ;
#19461=CARTESIAN_POINT ( 'NONE',  ( 206.2214737538543829, 104.7347325308398354, 45.00000000000000000 ) ) ;
#19462=CARTESIAN_POINT ( 'NONE',  ( 147.3660254037845334, 200.5814157129577779, -45.00000000000000000 ) ) ;
#19472=LINE ( 'NONE', #8276, #25784 ) ;
#19486=EDGE_LOOP ( 'NONE', ( #1421, #11710, #13549, #4986 ) ) ;
#19501=CARTESIAN_POINT ( 'NONE',  ( 150.5563491861040575, 203.0294372515228929, 45.00000000000000000 ) ) ;
#19531=DIRECTION ( 'NONE',  ( -0.9506505318133544602, -0.3102637045530566295, 0.000000000000000000 ) ) ;
#19540=ORIENTED_EDGE ( 'NONE', *, *, #11015, .T. ) ;
#19541=ORIENTED_EDGE ( 'NONE', *, *, #4873, .F. ) ;
#19543=EDGE_LOOP ( 'NONE', ( #20645, #9906, #26479, #24569 ) ) ;
#19569=ADVANCED_FACE ( 'NONE', ( #17548 ), #2037, .F. ) ;
#19589=CARTESIAN_POINT ( 'NONE',  ( 142.6536686473019699, 201.5224093497741649, -45.00000000000000000 ) ) ;
#19609=DIRECTION ( 'NONE',  ( 0.05364526231778203591, -0.9985600561963492439, 0.000000000000000000 ) ) ;
#19614=ORIENTED_EDGE ( 'NONE', *, *, #27460, .F. ) ;
#19635=DIRECTION ( 'NONE',  ( -0.05364526231779760679, -0.9985600561963485777, 0.000000000000000000 ) ) ;
#19640=DIRECTION ( 'NONE',  ( -0.000000000000000000, -0.000000000000000000, -1.000000000000000000 ) ) ;
#19642=ORIENTED_EDGE ( 'NONE', *, *, #9397, .T. ) ;
#19651=ORIENTED_EDGE ( 'NONE', *, *, #25383, .F. ) ;
#19663=VECTOR ( 'NONE', #5571, 1000.000000000000114 ) ;
#19688=ORIENTED_EDGE ( 'NONE', *, *, #16788, .F. ) ;
#19703=VERTEX_POINT ( 'NONE', #22858 ) ;
#19731=DIRECTION ( 'NONE',  ( -0.2588190451025286221, -0.9659258262890662028, 0.000000000000000000 ) ) ;
#19736=CARTESIAN_POINT ( 'NONE',  ( 144.9999999999998863, 220.0000000000000284, 45.00000000000000000 ) ) ;
#19766=DIRECTION ( 'NONE',  ( -0.9784193629480785193, 0.2066290158914672603, 0.000000000000000000 ) ) ;
#19789=EDGE_CURVE ( 'NONE', #4776, #3728, #2745, .T. ) ;
#19790=VERTEX_POINT ( 'NONE', #14249 ) ;
#19799=LINE ( 'NONE', #14937, #3561 ) ;
#19852=EDGE_CURVE ( 'NONE', #26795, #21098, #8336, .T. ) ;
#19927=PLANE ( 'NONE',  #7088 ) ;
#19959=PLANE ( 'NONE',  #18341 ) ;
#19969=VERTEX_POINT ( 'NONE', #8908 ) ;
#19996=DIRECTION ( 'NONE',  ( -0.9506505318133474658, 0.3102637045530776683, 0.000000000000000000 ) ) ;
#19999=VECTOR ( 'NONE', #16367, 1000.000000000000000 ) ;
#20020=CARTESIAN_POINT ( 'NONE',  ( -10.78991826960876033, 200.8449754580304898, -45.00000000000000000 ) ) ;
#20023=CARTESIAN_POINT ( 'NONE',  ( 203.1730087600953993, 54.44004362106413453, 45.00000000000000000 ) ) ;
#20030=DIRECTION ( 'NONE',  ( -0.2066290158914539099, 0.9784193629480814058, 0.000000000000000000 ) ) ;
#20033=LINE ( 'NONE', #15747, #23050 ) ;
#20044=ORIENTED_EDGE ( 'NONE', *, *, #12561, .F. ) ;
#20056=CARTESIAN_POINT ( 'NONE',  ( -58.76345596729049703, 58.76345596729049703, -45.00000000000000000 ) ) ;
#20077=ORIENTED_EDGE ( 'NONE', *, *, #9389, .T. ) ;
#20082=CARTESIAN_POINT ( 'NONE',  ( -51.90955279280624524, 193.7290884209386661, 45.00000000000000000 ) ) ;
#20114=AXIS2_PLACEMENT_3D ( 'NONE', #20162, #13284, #2198 ) ;
#20137=LINE ( 'NONE', #468, #10269 ) ;
#20152=VECTOR ( 'NONE', #718, 1000.000000000000114 ) ;
#20158=CARTESIAN_POINT ( 'NONE',  ( 137.6105238444012286, 200.1711027725236534, -45.00000000000000000 ) ) ;
#20162=CARTESIAN_POINT ( 'NONE',  ( 134.9999999999998579, 220.0000000000000284, 45.00000000000000000 ) ) ;
#20173=VECTOR ( 'NONE', #18352, 1000.000000000000000 ) ;
#20174=ORIENTED_EDGE ( 'NONE', *, *, #6271, .T. ) ;
#20179=CARTESIAN_POINT ( 'NONE',  ( -43.04748092857122543, 38.65804596583237895, 45.00000000000000000 ) ) ;
#20182=EDGE_CURVE ( 'NONE', #6540, #5518, #5013, .T. ) ;
#20183=ADVANCED_FACE ( 'NONE', ( #9195 ), #720, .F. ) ;
#20197=EDGE_CURVE ( 'NONE', #13479, #4776, #16098, .T. ) ;
#20218=ORIENTED_EDGE ( 'NONE', *, *, #25163, .T. ) ;
#20226=ADVANCED_FACE ( 'NONE', ( #18525 ), #22405, .F. ) ;
#20234=CARTESIAN_POINT ( 'NONE',  ( 184.7759657584203694, 39.02219989801907474, 45.00000000000000000 ) ) ;
#20238=CARTESIAN_POINT ( 'NONE',  ( 132.3894761555988282, 239.8288972274758919, -45.00000000000000000 ) ) ;
#20244=CARTESIAN_POINT ( 'NONE',  ( 203.1730087600953993, 54.44004362106413453, -45.00000000000000000 ) ) ;
#20255=AXIS2_PLACEMENT_3D ( 'NONE', #16651, #16376, #3133 ) ;
#20287=EDGE_CURVE ( 'NONE', #25781, #5376, #1791, .T. ) ;
#20290=PLANE ( 'NONE',  #17697 ) ;
#20296=DIRECTION ( 'NONE',  ( 1.000000000000000000, 0.000000000000000000, 0.000000000000000000 ) ) ;
#20315=DIRECTION ( 'NONE',  ( -0.3102637045530683979, 0.9506505318133506854, 0.000000000000000000 ) ) ;
#20326=ORIENTED_EDGE ( 'NONE', *, *, #3475, .F. ) ;
#20334=VERTEX_POINT ( 'NONE', #12875 ) ;
#20347=DIRECTION ( 'NONE',  ( 0.2588190451025252359, 0.9659258262890672020, -0.000000000000000000 ) ) ;
#20378=DIRECTION ( 'NONE',  ( 0.8916010070293484135, -0.4528218681382910060, 0.000000000000000000 ) ) ;
#20388=DIRECTION ( 'NONE',  ( -0.05364526231778204285, 0.9985600561963493549, 0.000000000000000000 ) ) ;
#20390=DIRECTION ( 'NONE',  ( -0.000000000000000000, -0.000000000000000000, -1.000000000000000000 ) ) ;
#20395=ADVANCED_FACE ( 'NONE', ( #3949 ), #25264, .F. ) ;
#20424=CARTESIAN_POINT ( 'NONE',  ( 115.5814157129579058, 207.6339745962153245, 45.00000000000000000 ) ) ;
#20430=VECTOR ( 'NONE', #25960, 1000.000000000000114 ) ;
#20435=ORIENTED_EDGE ( 'NONE', *, *, #21293, .T. ) ;
#20438=LINE ( 'NONE', #16140, #13029 ) ;
#20440=ORIENTED_EDGE ( 'NONE', *, *, #20956, .T. ) ;
#20458=CARTESIAN_POINT ( 'NONE',  ( -58.76345596729049703, 58.76345596729049703, 45.00000000000000000 ) ) ;
#20475=VERTEX_POINT ( 'NONE', #8977 ) ;
#20481=ADVANCED_FACE ( 'NONE', ( #13437 ), #4798, .F. ) ;
#20494=VECTOR ( 'NONE', #22165, 1000.000000000000114 ) ;
#20498=DIRECTION ( 'NONE',  ( 0.7440215159218921404, -0.6681556583950251094, 0.000000000000000000 ) ) ;
#20523=CARTESIAN_POINT ( 'NONE',  ( 121.6232796275294277, 239.4748271322486630, 45.00000000000000000 ) ) ;
#20546=EDGE_CURVE ( 'NONE', #19128, #12951, #15889, .T. ) ;
#20574=CARTESIAN_POINT ( 'NONE',  ( 135.1062353973271968, 7.258260926501912458, -45.00000000000000000 ) ) ;
#20593=CARTESIAN_POINT ( 'NONE',  ( 156.9574749595459195, 226.9187638636467739, 45.00000000000000000 ) ) ;
#20597=EDGE_CURVE ( 'NONE', #27997, #17680, #10996, .T. ) ;
#20604=CARTESIAN_POINT ( 'NONE',  ( 177.1897033089359184, 197.3087408678716770, -45.00000000000000000 ) ) ;
#20617=ORIENTED_EDGE ( 'NONE', *, *, #21127, .F. ) ;
#20620=EDGE_CURVE ( 'NONE', #19969, #860, #11721, .T. ) ;
#20630=DIRECTION ( 'NONE',  ( -0.05364526231779676024, -0.9985600561963485777, 0.000000000000000000 ) ) ;
#20632=CARTESIAN_POINT ( 'NONE',  ( -41.04971513216914047, 194.3765543069588659, 45.00000000000000000 ) ) ;
#20636=VECTOR ( 'NONE', #5567, 1000.000000000000000 ) ;
#20645=ORIENTED_EDGE ( 'NONE', *, *, #22190, .T. ) ;
#20647=EDGE_CURVE ( 'NONE', #4525, #26924, #18175, .T. ) ;
#20653=DIRECTION ( 'NONE',  ( -0.5457381880580733924, -0.8379557447115514313, 0.000000000000000000 ) ) ;
#20655=CARTESIAN_POINT ( 'NONE',  ( 124.3660254037843771, 240.4185842870417105, 45.00000000000000000 ) ) ;
#20656=CARTESIAN_POINT ( 'NONE',  ( -73.01279441628793165, 126.4618695315959087, -45.00000000000000000 ) ) ;
#20658=CARTESIAN_POINT ( 'NONE',  ( 184.7759657584203694, 39.02219989801907474, -45.00000000000000000 ) ) ;
#20668=EDGE_CURVE ( 'NONE', #20790, #14035, #649, .T. ) ;
#20703=CARTESIAN_POINT ( 'NONE',  ( 154.4185842870419663, 232.3660254037841639, -45.00000000000000000 ) ) ;
#20724=DIRECTION ( 'NONE',  ( -1.000000000000000000, 0.000000000000000000, 0.000000000000000000 ) ) ;
#20751=DIRECTION ( 'NONE',  ( -0.000000000000000000, -0.000000000000000000, -1.000000000000000000 ) ) ;
#20765=FACE_OUTER_BOUND ( 'NONE', #257, .T. ) ;
#20768=PLANE ( 'NONE',  #25076 ) ;
#20772=ORIENTED_EDGE ( 'NONE', *, *, #11870, .F. ) ;
#20777=ORIENTED_EDGE ( 'NONE', *, *, #3674, .F. ) ;
#20781=AXIS2_PLACEMENT_3D ( 'NONE', #15953, #2571, #7035 ) ;
#20785=ORIENTED_EDGE ( 'NONE', *, *, #28127, .T. ) ;
#20790=VERTEX_POINT ( 'NONE', #1621 ) ;
#20817=ORIENTED_EDGE ( 'NONE', *, *, #12160, .F. ) ;
#20819=ORIENTED_EDGE ( 'NONE', *, *, #21127, .T. ) ;
#20847=ORIENTED_EDGE ( 'NONE', *, *, #27423, .T. ) ;
#20850=ORIENTED_EDGE ( 'NONE', *, *, #14203, .F. ) ;
#20858=DIRECTION ( 'NONE',  ( -0.3102637045530707294, -0.9506505318133497973, 0.000000000000000000 ) ) ;
#20859=CARTESIAN_POINT ( 'NONE',  ( -15.28840184913744515, 9.956927649352207865, 45.00000000000000000 ) ) ;
#20864=VECTOR ( 'NONE', #14322, 1000.000000000000114 ) ;
#20869=DIRECTION ( 'NONE',  ( -0.4999999999999985012, 0.8660254037844394848, 0.000000000000000000 ) ) ;
#20870=DIRECTION ( 'NONE',  ( -0.000000000000000000, -0.000000000000000000, -1.000000000000000000 ) ) ;
#20872=CARTESIAN_POINT ( 'NONE',  ( 192.5108452903457419, 172.8810361401565672, 45.00000000000000000 ) ) ;
#20894=ORIENTED_EDGE ( 'NONE', *, *, #900, .T. ) ;
#20896=ORIENTED_EDGE ( 'NONE', *, *, #27460, .T. ) ;
#20927=ORIENTED_EDGE ( 'NONE', *, *, #894, .T. ) ;
#20930=VERTEX_POINT ( 'NONE', #11097 ) ;
#20955=EDGE_LOOP ( 'NONE', ( #12037, #19651, #27935, #10758 ) ) ;
#20956=EDGE_CURVE ( 'NONE', #16518, #25350, #8795, .T. ) ;
#20958=CARTESIAN_POINT ( 'NONE',  ( 141.9187638636469160, 241.9574749595457774, 45.00000000000000000 ) ) ;
#20963=ORIENTED_EDGE ( 'NONE', *, *, #2154, .T. ) ;
#20984=ORIENTED_EDGE ( 'NONE', *, *, #5867, .T. ) ;
#20989=DIRECTION ( 'NONE',  ( -0.000000000000000000, -0.000000000000000000, -1.000000000000000000 ) ) ;
#21009=VECTOR ( 'NONE', #4929, 1000.000000000000000 ) ;
#21022=EDGE_CURVE ( 'NONE', #5376, #20790, #20137, .T. ) ;
#21035=VECTOR ( 'NONE', #3687, 1000.000000000000000 ) ;
#21059=CARTESIAN_POINT ( 'NONE',  ( 115.5814157129579058, 207.6339745962153245, -45.00000000000000000 ) ) ;
#21062=CARTESIAN_POINT ( 'NONE',  ( 73.69623568533953062, -15.56365422765611051, -45.00000000000000000 ) ) ;
#21097=ORIENTED_EDGE ( 'NONE', *, *, #26038, .T. ) ;
#21098=VERTEX_POINT ( 'NONE', #22685 ) ;
#21107=CARTESIAN_POINT ( 'NONE',  ( -73.01279441628793165, 126.4618695315959087, 45.00000000000000000 ) ) ;
#21116=DIRECTION ( 'NONE',  ( 0.8379557447115549840, 0.5457381880580680633, 0.000000000000000000 ) ) ;
#21120=DIRECTION ( 'NONE',  ( -0.6681556583950251094, -0.7440215159218921404, 0.000000000000000000 ) ) ;
#21127=EDGE_CURVE ( 'NONE', #3496, #8917, #11638, .T. ) ;
#21142=VECTOR ( 'NONE', #21430, 1000.000000000000000 ) ;
#21144=DIRECTION ( 'NONE',  ( 0.3102637045530566295, -0.9506505318133544602, 0.000000000000000000 ) ) ;
#21145=LINE ( 'NONE', #3334, #12232 ) ;
#21147=EDGE_CURVE ( 'NONE', #11070, #14636, #13001, .T. ) ;
#21149=VECTOR ( 'NONE', #9792, 1000.000000000000000 ) ;
#21154=LINE ( 'NONE', #7287, #25719 ) ;
#21156=PLANE ( 'NONE',  #8464 ) ;
#21163=VERTEX_POINT ( 'NONE', #19589 ) ;
#21170=ORIENTED_EDGE ( 'NONE', *, *, #6986, .T. ) ;
#21183=CARTESIAN_POINT ( 'NONE',  ( 122.6339745962154808, 239.4185842870417389, 45.00000000000000000 ) ) ;
#21236=EDGE_LOOP ( 'NONE', ( #9231, #120, #4268, #9310 ) ) ;
#21249=DIRECTION ( 'NONE',  ( 0.2588190451025321748, 0.9659258262890653146, 0.000000000000000000 ) ) ;
#21265=VECTOR ( 'NONE', #18785, 1000.000000000000114 ) ;
#21269=AXIS2_PLACEMENT_3D ( 'NONE', #16201, #24949, #23076 ) ;
#21271=ADVANCED_FACE ( 'NONE', ( #4915, #26904 ), #7232, .T. ) ;
#21293=EDGE_CURVE ( 'NONE', #11731, #26795, #20438, .T. ) ;
#21298=LINE ( 'NONE', #6348, #10291 ) ;
#21304=ORIENTED_EDGE ( 'NONE', *, *, #12436, .F. ) ;
#21318=EDGE_CURVE ( 'NONE', #10728, #16518, #18426, .T. ) ;
#21332=FACE_OUTER_BOUND ( 'NONE', #19543, .T. ) ;
#21348=AXIS2_PLACEMENT_3D ( 'NONE', #6840, #15622, #19635 ) ;
#21365=VECTOR ( 'NONE', #14411, 1000.000000000000000 ) ;
#21368=DIRECTION ( 'NONE',  ( 0.8916010070293547418, 0.4528218681382786270, 0.000000000000000000 ) ) ;
#21386=EDGE_CURVE ( 'NONE', #2611, #3496, #16283, .T. ) ;
#21397=LINE ( 'NONE', #18962, #22714 ) ;
#21401=CARTESIAN_POINT ( 'NONE',  ( -48.38593899427829115, 148.2549133597845241, 45.00000000000000000 ) ) ;
#21422=ORIENTED_EDGE ( 'NONE', *, *, #12352, .T. ) ;
#21430=DIRECTION ( 'NONE',  ( -0.000000000000000000, -0.000000000000000000, -1.000000000000000000 ) ) ;
#21431=VERTEX_POINT ( 'NONE', #23298 ) ;
#21436=ORIENTED_EDGE ( 'NONE', *, *, #1339, .F. ) ;
#21464=DIRECTION ( 'NONE',  ( -0.000000000000000000, -0.000000000000000000, -1.000000000000000000 ) ) ;
#21480=CARTESIAN_POINT ( 'NONE',  ( 115.1711027725237528, 222.6105238444006886, -45.00000000000000000 ) ) ;
#21483=CARTESIAN_POINT ( 'NONE',  ( 112.5248869502488986, 215.0130877889307044, -45.00000000000000000 ) ) ;
#21492=ORIENTED_EDGE ( 'NONE', *, *, #14112, .F. ) ;
#21508=EDGE_CURVE ( 'NONE', #19969, #8240, #4172, .T. ) ;
#21534=VECTOR ( 'NONE', #9933, 1000.000000000000000 ) ;
#21538=DIRECTION ( 'NONE',  ( -0.05364526231776645809, 0.9985600561963501320, 0.000000000000000000 ) ) ;
#21558=VERTEX_POINT ( 'NONE', #9174 ) ;
#21577=ADVANCED_FACE ( 'NONE', ( #4991 ), #6870, .F. ) ;
#21587=CARTESIAN_POINT ( 'NONE',  ( 134.9999999999998579, 220.0000000000000284, -45.00000000000000000 ) ) ;
#21599=EDGE_CURVE ( 'NONE', #13260, #11332, #13493, .T. ) ;
#21617=DIRECTION ( 'NONE',  ( 1.000000000000000000, 0.000000000000000000, 0.000000000000000000 ) ) ;
#21686=CARTESIAN_POINT ( 'NONE',  ( 156.9574749595459195, 226.9187638636467739, -45.00000000000000000 ) ) ;
#21695=EDGE_LOOP ( 'NONE', ( #26891, #11140, #13035, #23632 ) ) ;
#21705=FACE_OUTER_BOUND ( 'NONE', #1945, .T. ) ;
#21706=EDGE_LOOP ( 'NONE', ( #3850, #1102, #6952, #6370 ) ) ;
#21731=DIRECTION ( 'NONE',  ( -0.000000000000000000, -0.000000000000000000, -1.000000000000000000 ) ) ;
#21795=FACE_OUTER_BOUND ( 'NONE', #15776, .T. ) ;
#21814=AXIS2_PLACEMENT_3D ( 'NONE', #9799, #12244, #18278 ) ;
#21819=DIRECTION ( 'NONE',  ( -0.000000000000000000, -0.000000000000000000, -1.000000000000000000 ) ) ;
#21820=EDGE_CURVE ( 'NONE', #7097, #5376, #19201, .T. ) ;
#21841=ORIENTED_EDGE ( 'NONE', *, *, #7733, .T. ) ;
#21863=ORIENTED_EDGE ( 'NONE', *, *, #28127, .F. ) ;
#21866=DIRECTION ( 'NONE',  ( 0.8660254037844394848, -0.4999999999999985012, 0.000000000000000000 ) ) ;
#21880=VERTEX_POINT ( 'NONE', #24797 ) ;
#21890=DIRECTION ( 'NONE',  ( -0.3102637045530777238, -0.9506505318133475768, 0.000000000000000000 ) ) ;
#21909=CARTESIAN_POINT ( 'NONE',  ( 130.0130877889309602, 242.4751130497508029, 45.00000000000000000 ) ) ;
#21910=DIRECTION ( 'NONE',  ( 0.7071067811865474617, -0.7071067811865474617, 0.000000000000000000 ) ) ;
#21927=DIRECTION ( 'NONE',  ( 0.2588190451025121908, -0.9659258262890705327, 0.000000000000000000 ) ) ;
#21931=CARTESIAN_POINT ( 'NONE',  ( 115.5814157129578916, 232.3660254037840502, 45.00000000000000000 ) ) ;
#21932=LINE ( 'NONE', #20056, #20430 ) ;
#21944=ORIENTED_EDGE ( 'NONE', *, *, #19789, .T. ) ;
#21958=LINE ( 'NONE', #15083, #6134 ) ;
#21962=CARTESIAN_POINT ( 'NONE',  ( 158.7404207507997853, 42.53436754635193040, 45.00000000000000000 ) ) ;
#21973=ORIENTED_EDGE ( 'NONE', *, *, #6073, .F. ) ;
#21983=CARTESIAN_POINT ( 'NONE',  ( 145.6339745962156940, 199.5814157129578064, 45.00000000000000000 ) ) ;
#21995=VECTOR ( 'NONE', #22548, 1000.000000000000000 ) ;
#21996=CARTESIAN_POINT ( 'NONE',  ( 150.5563491861040575, 203.0294372515228929, 45.00000000000000000 ) ) ;
#22008=VECTOR ( 'NONE', #2666, 1000.000000000000000 ) ;
#22010=CARTESIAN_POINT ( 'NONE',  ( 216.4313787033304379, 124.9567147554451623, -45.00000000000000000 ) ) ;
#22014=ORIENTED_EDGE ( 'NONE', *, *, #13137, .T. ) ;
#22020=EDGE_LOOP ( 'NONE', ( #20819, #13062, #17279, #20174 ) ) ;
#22026=CARTESIAN_POINT ( 'NONE',  ( 206.2214737538543829, 104.7347325308398354, -45.00000000000000000 ) ) ;
#22032=CARTESIAN_POINT ( 'NONE',  ( 8.415662294793918363, -4.274104551145060604, -45.00000000000000000 ) ) ;
#22038=CARTESIAN_POINT ( 'NONE',  ( 128.0812361363527998, 241.9574749595457774, -45.00000000000000000 ) ) ;
#22079=DIRECTION ( 'NONE',  ( -0.9506505318133506854, -0.3102637045530683979, 0.000000000000000000 ) ) ;
#22088=ORIENTED_EDGE ( 'NONE', *, *, #3639, .T. ) ;
#22094=ORIENTED_EDGE ( 'NONE', *, *, #7486, .F. ) ;
#22104=CARTESIAN_POINT ( 'NONE',  ( 137.6105238444012286, 200.1711027725236534, 45.00000000000000000 ) ) ;
#22106=FACE_OUTER_BOUND ( 'NONE', #13098, .T. ) ;
#22120=PRODUCT_DEFINITION_FORMATION_WITH_SPECIFIED_SOURCE ( 'ANY', '', #6610, .NOT_KNOWN. ) ;
#22152=AXIS2_PLACEMENT_3D ( 'NONE', #23924, #5583, #19609 ) ;
#22153=CARTESIAN_POINT ( 'NONE',  ( 81.39309752945497678, 249.3891174404998594, 45.00000000000000000 ) ) ;
#22164=VERTEX_POINT ( 'NONE', #20158 ) ;
#22165=DIRECTION ( 'NONE',  ( -0.9985600561963481336, 0.05364526231780537141, 0.000000000000000000 ) ) ;
#22167=ORIENTED_EDGE ( 'NONE', *, *, #12972, .T. ) ;
#22170=DIRECTION ( 'NONE',  ( -0.4528218681382909505, -0.8916010070293484135, 0.000000000000000000 ) ) ;
#22180=DIRECTION ( 'NONE',  ( -0.000000000000000000, -0.000000000000000000, -1.000000000000000000 ) ) ;
#22189=ORIENTED_EDGE ( 'NONE', *, *, #16297, .T. ) ;
#22190=EDGE_CURVE ( 'NONE', #627, #860, #9101, .T. ) ;
#22203=ADVANCED_FACE ( 'NONE', ( #11113 ), #4630, .F. ) ;
#22220=CARTESIAN_POINT ( 'NONE',  ( 141.9187638636469160, 241.9574749595457774, -45.00000000000000000 ) ) ;
#22221=CARTESIAN_POINT ( 'NONE',  ( 136.0000000000000853, 196.9999999999997442, -45.00000000000000000 ) ) ;
#22236=VERTEX_POINT ( 'NONE', #16561 ) ;
#22247=CARTESIAN_POINT ( 'NONE',  ( 147.1752285801744904, 204.1329331941753082, 45.00000000000000000 ) ) ;
#22258=CARTESIAN_POINT ( 'NONE',  ( 153.4775906502255509, 227.6536686473015436, 45.00000000000000000 ) ) ;
#22282=PLANE ( 'NONE',  #23829 ) ;
#22321=VECTOR ( 'NONE', #20630, 1000.000000000000114 ) ;
#22322=CARTESIAN_POINT ( 'NONE',  ( 113.0425250404539241, 213.0812361363525440, 45.00000000000000000 ) ) ;
#22327=DIRECTION ( 'NONE',  ( -0.000000000000000000, -0.000000000000000000, -1.000000000000000000 ) ) ;
#22356=ADVANCED_FACE ( 'NONE', ( #10094 ), #10516, .F. ) ;
#22367=DIRECTION ( 'NONE',  ( 0.2066290158914539099, -0.9784193629480814058, 0.000000000000000000 ) ) ;
#22371=DIRECTION ( 'NONE',  ( -0.5457381880580733924, -0.8379557447115514313, 0.000000000000000000 ) ) ;
#22379=VECTOR ( 'NONE', #12649, 1000.000000000000227 ) ;
#22401=CARTESIAN_POINT ( 'NONE',  ( 93.17300876009500143, -24.96563245364655259, 45.00000000000000000 ) ) ;
#22405=PLANE ( 'NONE',  #17553 ) ;
#22415=CARTESIAN_POINT ( 'NONE',  ( 134.6436608991879496, 206.7391133850113079, 45.00000000000000000 ) ) ;
#22418=ORIENTED_EDGE ( 'NONE', *, *, #7465, .F. ) ;
#22469=ORIENTED_EDGE ( 'NONE', *, *, #17747, .F. ) ;
#22485=VERTEX_POINT ( 'NONE', #10236 ) ;
#22498=VERTEX_POINT ( 'NONE', #27872 ) ;
#22501=EDGE_CURVE ( 'NONE', #3649, #14719, #8216, .T. ) ;
#22506=DIRECTION ( 'NONE',  ( -0.6681556583950049033, 0.7440215159219103480, 0.000000000000000000 ) ) ;
#22515=DIRECTION ( 'NONE',  ( -0.000000000000000000, -0.000000000000000000, -1.000000000000000000 ) ) ;
#22529=ORIENTED_EDGE ( 'NONE', *, *, #8651, .F. ) ;
#22540=LINE ( 'NONE', #3410, #10830 ) ;
#22548=DIRECTION ( 'NONE',  ( -0.9659258262890662028, 0.2588190451025286221, 0.000000000000000000 ) ) ;
#22551=ORIENTED_EDGE ( 'NONE', *, *, #12060, .F. ) ;
#22616=ORIENTED_EDGE ( 'NONE', *, *, #26222, .F. ) ;
#22640=ORIENTED_EDGE ( 'NONE', *, *, #20182, .F. ) ;
#22646=ORIENTED_EDGE ( 'NONE', *, *, #21508, .T. ) ;
#22658=FACE_OUTER_BOUND ( 'NONE', #17850, .T. ) ;
#22668=EDGE_LOOP ( 'NONE', ( #19540, #24859, #18256, #21170 ) ) ;
#22685=CARTESIAN_POINT ( 'NONE',  ( 119.4436508138959567, 203.0294372515225518, 45.00000000000000000 ) ) ;
#22714=VECTOR ( 'NONE', #25987, 1000.000000000000000 ) ;
#22734=VECTOR ( 'NONE', #10015, 1000.000000000000114 ) ;
#22756=EDGE_CURVE ( 'NONE', #8677, #11330, #599, .T. ) ;
#22777=ORIENTED_EDGE ( 'NONE', *, *, #7156, .F. ) ;
#22790=EDGE_CURVE ( 'NONE', #4583, #23257, #17082, .T. ) ;
#22798=DIRECTION ( 'NONE',  ( -0.000000000000000000, -0.000000000000000000, -1.000000000000000000 ) ) ;
#22816=LINE ( 'NONE', #1115, #6308 ) ;
#22847=EDGE_CURVE ( 'NONE', #7652, #10728, #12369, .T. ) ;
#22858=CARTESIAN_POINT ( 'NONE',  ( 153.4775906502256930, 212.3463313526982859, 45.00000000000000000 ) ) ;
#22862=VECTOR ( 'NONE', #5401, 999.9999999999998863 ) ;
#22868=ORIENTED_EDGE ( 'NONE', *, *, #16649, .T. ) ;
#22871=CARTESIAN_POINT ( 'NONE',  ( 122.6339745962156229, 200.5814157129576074, 45.00000000000000000 ) ) ;
#22872=ORIENTED_EDGE ( 'NONE', *, *, #27628, .F. ) ;
#22886=CYLINDRICAL_SURFACE ( 'NONE', #10839, 10.00000000000000888 ) ;
#22895=DIRECTION ( 'NONE',  ( 0.7071067811865475727, -0.7071067811865475727, 0.000000000000000000 ) ) ;
#22898=DIRECTION ( 'NONE',  ( -0.8916010070293547418, -0.4528218681382785715, 0.000000000000000000 ) ) ;
#22905=VECTOR ( 'NONE', #27870, 1000.000000000000114 ) ;
#22906=CARTESIAN_POINT ( 'NONE',  ( 119.4436508138957720, 236.9705627484767376, -45.00000000000000000 ) ) ;
#22908=EDGE_CURVE ( 'NONE', #21163, #25781, #17786, .T. ) ;
#22912=ORIENTED_EDGE ( 'NONE', *, *, #28284, .T. ) ;
#22915=AXIS2_PLACEMENT_3D ( 'NONE', #15509, #24399, #24123 ) ;
#22916=EDGE_CURVE ( 'NONE', #25350, #24989, #21958, .T. ) ;
#22927=VECTOR ( 'NONE', #2968, 1000.000000000000000 ) ;
#22934=DIRECTION ( 'NONE',  ( 0.3102637045530683979, -0.9506505318133506854, 0.000000000000000000 ) ) ;
#22938=DIRECTION ( 'NONE',  ( 0.4528218681382754074, -0.8916010070293562961, 0.000000000000000000 ) ) ;
#22951=ORIENTED_EDGE ( 'NONE', *, *, #10922, .F. ) ;
#22969=VERTEX_POINT ( 'NONE', #26124 ) ;
#22985=VERTEX_POINT ( 'NONE', #15653 ) ;
#22986=CARTESIAN_POINT ( 'NONE',  ( 157.6866818850739662, 8.471341669691319964, 45.00000000000000000 ) ) ;
#22997=CARTESIAN_POINT ( 'NONE',  ( 124.3660254037845192, 199.5814157129575506, 45.00000000000000000 ) ) ;
#23011=EDGE_LOOP ( 'NONE', ( #4652, #27939, #27895, #10859 ) ) ;
#23014=AXIS2_PLACEMENT_3D ( 'NONE', #20458, #22895, #781 ) ;
#23032=PLANE ( 'NONE',  #11874 ) ;
#23036=ORIENTED_EDGE ( 'NONE', *, *, #11870, .T. ) ;
#23039=EDGE_CURVE ( 'NONE', #7688, #22164, #17649, .T. ) ;
#23044=ORIENTED_EDGE ( 'NONE', *, *, #12998, .F. ) ;
#23048=ORIENTED_EDGE ( 'NONE', *, *, #5240, .F. ) ;
#23050=VECTOR ( 'NONE', #4239, 1000.000000000000000 ) ;
#23055=CARTESIAN_POINT ( 'NONE',  ( 157.4751130497510303, 215.0130877889310455, 45.00000000000000000 ) ) ;
#23070=CARTESIAN_POINT ( 'NONE',  ( 122.6339745962154808, 239.4185842870417389, -45.00000000000000000 ) ) ;
#23076=DIRECTION ( 'NONE',  ( 0.000000000000000000, -0.000000000000000000, 1.000000000000000000 ) ) ;
#23077=EDGE_LOOP ( 'NONE', ( #24646, #15437, #15853, #17348 ) ) ;
#23083=CARTESIAN_POINT ( 'NONE',  ( -73.01279441628793165, 126.4618695315959087, 45.00000000000000000 ) ) ;
#23094=VERTEX_POINT ( 'NONE', #561 ) ;
#23096=ORIENTED_EDGE ( 'NONE', *, *, #5580, .T. ) ;
#23101=VECTOR ( 'NONE', #26266, 1000.000000000000114 ) ;
#23110=DIRECTION ( 'NONE',  ( 0.4528218681382786270, -0.8916010070293547418, 0.000000000000000000 ) ) ;
#23141=EDGE_CURVE ( 'NONE', #26924, #2611, #2845, .T. ) ;
#23148=FACE_OUTER_BOUND ( 'NONE', #19486, .T. ) ;
#23161=LINE ( 'NONE', #25583, #22905 ) ;
#23162=ORIENTED_EDGE ( 'NONE', *, *, #5240, .T. ) ;
#23169=CARTESIAN_POINT ( 'NONE',  ( 141.9187638636471434, 198.0425250404537678, 45.00000000000000000 ) ) ;
#23196=LINE ( 'NONE', #25347, #7660 ) ;
#23200=VECTOR ( 'NONE', #24943, 1000.000000000000000 ) ;
#23228=PLANE ( 'NONE',  #4816 ) ;
#23249=DIRECTION ( 'NONE',  ( 0.8916010070293562961, 0.4528218681382754629, -0.000000000000000000 ) ) ;
#23253=EDGE_CURVE ( 'NONE', #3880, #21558, #28336, .T. ) ;
#23257=VERTEX_POINT ( 'NONE', #19312 ) ;
#23258=DIRECTION ( 'NONE',  ( -0.9506505318133544602, -0.3102637045530566295, 0.000000000000000000 ) ) ;
#23298=CARTESIAN_POINT ( 'NONE',  ( 132.3894761555990556, 200.1711027725235397, -45.00000000000000000 ) ) ;
#23317=FACE_OUTER_BOUND ( 'NONE', #9282, .T. ) ;
#23337=EDGE_CURVE ( 'NONE', #18077, #4836, #4922, .T. ) ;
#23352=PLANE ( 'NONE',  #21269 ) ;
#23358=ORIENTED_EDGE ( 'NONE', *, *, #25514, .F. ) ;
#23379=LINE ( 'NONE', #12056, #21035 ) ;
#23385=CARTESIAN_POINT ( 'NONE',  ( 74.37710191228967460, 227.8920494084358950, 45.00000000000000000 ) ) ;
#23402=ORIENTED_EDGE ( 'NONE', *, *, #17543, .T. ) ;
#23410=CARTESIAN_POINT ( 'NONE',  ( 134.0000000000000853, 196.9999999999997442, 45.00000000000000000 ) ) ;
#23438=ORIENTED_EDGE ( 'NONE', *, *, #894, .F. ) ;
#23443=DIRECTION ( 'NONE',  ( -0.5000000000000106581, -0.8660254037844326014, 0.000000000000000000 ) ) ;
#23455=CARTESIAN_POINT ( 'NONE',  ( -48.38593899427829115, 148.2549133597845241, 45.00000000000000000 ) ) ;
#23468=CARTESIAN_POINT ( 'NONE',  ( 139.9869122110687840, 242.4751130497508314, -45.00000000000000000 ) ) ;
#23469=CARTESIAN_POINT ( 'NONE',  ( 113.0425250404538673, 226.9187638636466602, 45.00000000000000000 ) ) ;
#23488=VECTOR ( 'NONE', #16438, 1000.000000000000000 ) ;
#23494=CARTESIAN_POINT ( 'NONE',  ( -26.23654403271235225, 26.23654403271337543, 45.00000000000000000 ) ) ;
#23502=LINE ( 'NONE', #3953, #8363 ) ;
#23506=DIRECTION ( 'NONE',  ( 0.2588190451025286221, 0.9659258262890662028, 0.000000000000000000 ) ) ;
#23507=VERTEX_POINT ( 'NONE', #1048 ) ;
#23531=VECTOR ( 'NONE', #12960, 1000.000000000000000 ) ;
#23568=ADVANCED_FACE ( 'NONE', ( #18438 ), #27189, .F. ) ;
#23575=ORIENTED_EDGE ( 'NONE', *, *, #9389, .F. ) ;
#23577=PLANE ( 'NONE',  #2580 ) ;
#23586=DIRECTION ( 'NONE',  ( 0.3102637045530707294, 0.9506505318133497973, 0.000000000000000000 ) ) ;
#23590=DIRECTION ( 'NONE',  ( -0.9659258262890670910, -0.2588190451025251804, 0.000000000000000000 ) ) ;
#23608=ORIENTED_EDGE ( 'NONE', *, *, #13669, .F. ) ;
#23613=VECTOR ( 'NONE', #22371, 1000.000000000000114 ) ;
#23632=ORIENTED_EDGE ( 'NONE', *, *, #16547, .T. ) ;
#23660=LINE ( 'NONE', #26084, #18776 ) ;
#23662=ADVANCED_FACE ( 'NONE', ( #23875 ), #12546, .F. ) ;
#23672=DIRECTION ( 'NONE',  ( 0.9784193629480828491, 0.2066290158914464437, 0.000000000000000000 ) ) ;
#23695=ADVANCED_FACE ( 'NONE', ( #3756 ), #1606, .F. ) ;
#23708=VECTOR ( 'NONE', #3928, 999.9999999999998863 ) ;
#23719=ORIENTED_EDGE ( 'NONE', *, *, #1466, .F. ) ;
#23737=CARTESIAN_POINT ( 'NONE',  ( 204.8742559748123426, 133.4291290931197977, 45.00000000000000000 ) ) ;
#23738=ORIENTED_EDGE ( 'NONE', *, *, #20597, .F. ) ;
#23748=ORIENTED_EDGE ( 'NONE', *, *, #3666, .T. ) ;
#23755=DIRECTION ( 'NONE',  ( 0.4528218681383003319, 0.8916010070293436396, 0.000000000000000000 ) ) ;
#23756=ORIENTED_EDGE ( 'NONE', *, *, #27072, .F. ) ;
#23769=ORIENTED_EDGE ( 'NONE', *, *, #15337, .T. ) ;
#23774=LINE ( 'NONE', #15169, #15328 ) ;
#23783=DIRECTION ( 'NONE',  ( 0.9659258262890670910, -0.2588190451025251804, 0.000000000000000000 ) ) ;
#23798=VERTEX_POINT ( 'NONE', #21996 ) ;
#23829=AXIS2_PLACEMENT_3D ( 'NONE', #2592, #15836, #4889 ) ;
#23866=EDGE_LOOP ( 'NONE', ( #20777, #1636 ) ) ;
#23875=FACE_OUTER_BOUND ( 'NONE', #8168, .T. ) ;
#23910=DIRECTION ( 'NONE',  ( -0.000000000000000000, -0.000000000000000000, -1.000000000000000000 ) ) ;
#23924=CARTESIAN_POINT ( 'NONE',  ( 157.6866818850739662, 8.471341669691319964, 45.00000000000000000 ) ) ;
#23931=EDGE_CURVE ( 'NONE', #13241, #27691, #12090, .T. ) ;
#23933=VERTEX_POINT ( 'NONE', #25283 ) ;
#23974=ORIENTED_EDGE ( 'NONE', *, *, #23141, .F. ) ;
#23977=DIRECTION ( 'NONE',  ( -0.000000000000000000, 0.000000000000000000, 1.000000000000000000 ) ) ;
#24016=ORIENTED_EDGE ( 'NONE', *, *, #20197, .F. ) ;
#24023=VECTOR ( 'NONE', #1426, 1000.000000000000227 ) ;
#24032=ORIENTED_EDGE ( 'NONE', *, *, #13486, .F. ) ;
#24037=( NAMED_UNIT ( * ) PLANE_ANGLE_UNIT ( ) SI_UNIT ( $, .RADIAN. ) );
#24053=EDGE_CURVE ( 'NONE', #10285, #25999, #28132, .T. ) ;
#24072=CARTESIAN_POINT ( 'NONE',  ( 122.6339745962156229, 200.5814157129576074, 45.00000000000000000 ) ) ;
#24095=CARTESIAN_POINT ( 'NONE',  ( 122.6339745962154808, 239.4185842870417389, 45.00000000000000000 ) ) ;
#24113=EDGE_CURVE ( 'NONE', #8240, #22485, #21397, .T. ) ;
#24114=CARTESIAN_POINT ( 'NONE',  ( 192.5108452903457419, 172.8810361401565672, -45.00000000000000000 ) ) ;
#24120=VERTEX_POINT ( 'NONE', #12510 ) ;
#24123=DIRECTION ( 'NONE',  ( 0.2066290158914688702, 0.9784193629480781862, 0.000000000000000000 ) ) ;
#24141=ORIENTED_EDGE ( 'NONE', *, *, #16297, .F. ) ;
#24234=VERTEX_POINT ( 'NONE', #28273 ) ;
#24245=ADVANCED_FACE ( 'NONE', ( #26129 ), #15809, .F. ) ;
#24258=DIRECTION ( 'NONE',  ( -0.000000000000000000, -0.000000000000000000, -1.000000000000000000 ) ) ;
#24262=DIRECTION ( 'NONE',  ( -0.2588190451025121908, 0.9659258262890705327, 0.000000000000000000 ) ) ;
#24265=PLANE ( 'NONE',  #27861 ) ;
#24278=ORIENTED_EDGE ( 'NONE', *, *, #12998, .T. ) ;
#24288=DIRECTION ( 'NONE',  ( 0.7440215159219069063, 0.6681556583950086781, 0.000000000000000000 ) ) ;
#24304=ORIENTED_EDGE ( 'NONE', *, *, #26114, .T. ) ;
#24330=DIRECTION ( 'NONE',  ( -0.8379557447115656421, -0.5457381880580516320, 0.000000000000000000 ) ) ;
#24334=FACE_OUTER_BOUND ( 'NONE', #12350, .T. ) ;
#24350=VERTEX_POINT ( 'NONE', #2850 ) ;
#24368=ADVANCED_FACE ( 'NONE', ( #7315 ), #24841, .F. ) ;
#24375=DIRECTION ( 'NONE',  ( -0.000000000000000000, -0.000000000000000000, -1.000000000000000000 ) ) ;
#24377=LINE ( 'NONE', #686, #22927 ) ;
#24389=ORIENTED_EDGE ( 'NONE', *, *, #6137, .T. ) ;
#24394=CARTESIAN_POINT ( 'NONE',  ( 0.000000000000000000, 242.9999999999997158, 45.00000000000000000 ) ) ;
#24399=DIRECTION ( 'NONE',  ( 0.9784193629480781862, -0.2066290158914688702, 0.000000000000000000 ) ) ;
#24402=CARTESIAN_POINT ( 'NONE',  ( 137.6105238444007455, 239.8288972274759203, 45.00000000000000000 ) ) ;
#24403=DIRECTION ( 'NONE',  ( 0.9659258262890706437, 0.2588190451025122463, -0.000000000000000000 ) ) ;
#24407=LINE ( 'NONE', #24843, #2192 ) ;
#24417=EDGE_LOOP ( 'NONE', ( #27234, #6016, #24141, #16552 ) ) ;
#24430=ORIENTED_EDGE ( 'NONE', *, *, #10922, .T. ) ;
#24433=EDGE_CURVE ( 'NONE', #9062, #27691, #17057, .T. ) ;
#24466=CARTESIAN_POINT ( 'NONE',  ( 111.5363082892543218, -5.992022692082500157, 45.00000000000000000 ) ) ;
#24471=CARTESIAN_POINT ( 'NONE',  ( 28.57744295357075259, -14.51376905457599342, 45.00000000000000000 ) ) ;
#24493=PLANE ( 'NONE',  #1885 ) ;
#24505=LINE ( 'NONE', #4811, #10402 ) ;
#24509=ORIENTED_EDGE ( 'NONE', *, *, #6690, .T. ) ;
#24522=LINE ( 'NONE', #17628, #17112 ) ;
#24532=EDGE_CURVE ( 'NONE', #8917, #26858, #21932, .T. ) ;
#24555=PLANE ( 'NONE',  #17087 ) ;
#24569=ORIENTED_EDGE ( 'NONE', *, *, #7156, .T. ) ;
#24587=ORIENTED_EDGE ( 'NONE', *, *, #14550, .F. ) ;
#24626=LINE ( 'NONE', #2779, #25136 ) ;
#24645=ORIENTED_EDGE ( 'NONE', *, *, #14238, .F. ) ;
#24646=ORIENTED_EDGE ( 'NONE', *, *, #10137, .T. ) ;
#24656=VECTOR ( 'NONE', #7051, 1000.000000000000000 ) ;
#24660=LINE ( 'NONE', #3092, #9287 ) ;
#24670=CARTESIAN_POINT ( 'NONE',  ( 197.6424708188942816, 64.50455043276784295, 45.00000000000000000 ) ) ;
#24711=ORIENTED_EDGE ( 'NONE', *, *, #7442, .T. ) ;
#24733=ADVANCED_FACE ( 'NONE', ( #951 ), #9150, .F. ) ;
#24740=LINE ( 'NONE', #12100, #4777 ) ;
#24750=FACE_OUTER_BOUND ( 'NONE', #7509, .T. ) ;
#24762=EDGE_CURVE ( 'NONE', #12951, #2873, #10157, .T. ) ;
#24769=VERTEX_POINT ( 'NONE', #12464 ) ;
#24773=PLANE ( 'NONE',  #23014 ) ;
#24789=LINE ( 'NONE', #9276, #18161 ) ;
#24796=ORIENTED_EDGE ( 'NONE', *, *, #4655, .T. ) ;
#24797=CARTESIAN_POINT ( 'NONE',  ( 115.5814157129578916, 232.3660254037840502, -45.00000000000000000 ) ) ;
#24813=VECTOR ( 'NONE', #5109, 1000.000000000000000 ) ;
#24825=ADVANCED_FACE ( 'NONE', ( #27936 ), #23228, .F. ) ;
#24830=CARTESIAN_POINT ( 'NONE',  ( 156.9574749595459764, 213.0812361363529988, 45.00000000000000000 ) ) ;
#24841=PLANE ( 'NONE',  #716 ) ;
#24843=CARTESIAN_POINT ( 'NONE',  ( 121.6232796275294277, 239.4748271322486630, 45.00000000000000000 ) ) ;
#24845=DIRECTION ( 'NONE',  ( 0.4999999999999985012, -0.8660254037844394848, 0.000000000000000000 ) ) ;
#24859=ORIENTED_EDGE ( 'NONE', *, *, #28284, .F. ) ;
#24864=CARTESIAN_POINT ( 'NONE',  ( 47.90501010967909679, 226.8374036014029969, -45.00000000000000000 ) ) ;
#24865=ADVANCED_FACE ( 'NONE', ( #12324 ), #3531, .F. ) ;
#24877=ORIENTED_EDGE ( 'NONE', *, *, #25514, .T. ) ;
#24887=ORIENTED_EDGE ( 'NONE', *, *, #2401, .T. ) ;
#24894=EDGE_CURVE ( 'NONE', #7688, #9244, #6403, .T. ) ;
#24906=VECTOR ( 'NONE', #8292, 1000.000000000000000 ) ;
#24909=VERTEX_POINT ( 'NONE', #11144 ) ;
#24913=DIRECTION ( 'NONE',  ( 0.9506505318133544602, 0.3102637045530566295, 0.000000000000000000 ) ) ;
#24915=ORIENTED_EDGE ( 'NONE', *, *, #17613, .F. ) ;
#24920=ORIENTED_EDGE ( 'NONE', *, *, #20668, .F. ) ;
#24943=DIRECTION ( 'NONE',  ( -0.7071067811865336949, 0.7071067811865613395, 0.000000000000000000 ) ) ;
#24949=DIRECTION ( 'NONE',  ( 0.000000000000000000, 1.000000000000000000, 0.000000000000000000 ) ) ;
#24951=VECTOR ( 'NONE', #8180, 1000.000000000000000 ) ;
#24954=CARTESIAN_POINT ( 'NONE',  ( 114.5814157129578916, 209.3660254037841923, -45.00000000000000000 ) ) ;
#24957=ORIENTED_EDGE ( 'NONE', *, *, #12521, .T. ) ;
#24989=VERTEX_POINT ( 'NONE', #15326 ) ;
#24995=ORIENTED_EDGE ( 'NONE', *, *, #16083, .F. ) ;
#24996=DIRECTION ( 'NONE',  ( -0.8379557447115515423, 0.5457381880580733924, 0.000000000000000000 ) ) ;
#25008=CARTESIAN_POINT ( 'NONE',  ( -66.26041567618258910, 130.4659900502583127, -45.00000000000000000 ) ) ;
#25028=EDGE_LOOP ( 'NONE', ( #5085, #6362, #17399, #2189 ) ) ;
#25040=CARTESIAN_POINT ( 'NONE',  ( 141.9187638636471434, 198.0425250404537678, -45.00000000000000000 ) ) ;
#25051=ORIENTED_EDGE ( 'NONE', *, *, #22756, .T. ) ;
#25058=DIRECTION ( 'NONE',  ( -0.2066290158914688424, -0.9784193629480781862, 0.000000000000000000 ) ) ;
#25059=EDGE_CURVE ( 'NONE', #4836, #8677, #24789, .T. ) ;
#25065=CARTESIAN_POINT ( 'NONE',  ( 0.000000000000000000, 0.000000000000000000, 0.000000000000000000 ) ) ;
#25076=AXIS2_PLACEMENT_3D ( 'NONE', #11886, #20347, #2814 ) ;
#25086=CARTESIAN_POINT ( 'NONE',  ( 206.2214737538543829, 104.7347325308398354, 45.00000000000000000 ) ) ;
#25094=DIRECTION ( 'NONE',  ( 0.8660254037844455910, 0.4999999999999881206, 0.000000000000000000 ) ) ;
#25095=ORIENTED_EDGE ( 'NONE', *, *, #27281, .F. ) ;
#25115=DIRECTION ( 'NONE',  ( -0.4528218681382754629, 0.8916010070293562961, 0.000000000000000000 ) ) ;
#25116=DIRECTION ( 'NONE',  ( -0.9506505318133482429, 0.3102637045530752813, 0.000000000000000000 ) ) ;
#25119=LINE ( 'NONE', #9338, #20152 ) ;
#25127=ORIENTED_EDGE ( 'NONE', *, *, #13321, .T. ) ;
#25132=LINE ( 'NONE', #22986, #11060 ) ;
#25136=VECTOR ( 'NONE', #7390, 1000.000000000000000 ) ;
#25163=EDGE_CURVE ( 'NONE', #20475, #21163, #5665, .T. ) ;
#25166=DIRECTION ( 'NONE',  ( -0.000000000000000000, 0.000000000000000000, 1.000000000000000000 ) ) ;
#25168=CARTESIAN_POINT ( 'NONE',  ( 111.9999999999968878, -1.554312234475174324E-12, 45.00000000000000000 ) ) ;
#25170=FACE_OUTER_BOUND ( 'NONE', #15363, .T. ) ;
#25181=CARTESIAN_POINT ( 'NONE',  ( 113.0425250404538673, 226.9187638636466602, -45.00000000000000000 ) ) ;
#25193=LINE ( 'NONE', #20604, #15386 ) ;
#25199=VECTOR ( 'NONE', #24845, 1000.000000000000114 ) ;
#25209=EDGE_CURVE ( 'NONE', #23933, #18077, #14718, .T. ) ;
#25217=AXIS2_PLACEMENT_3D ( 'NONE', #17734, #15597, #20030 ) ;
#25222=LINE ( 'NONE', #14048, #3123 ) ;
#25228=CARTESIAN_POINT ( 'NONE',  ( 111.5363082892543218, -5.992022692082500157, 45.00000000000000000 ) ) ;
#25259=CARTESIAN_POINT ( 'NONE',  ( 111.9999999999999574, 220.9999999999996874, -45.00000000000000000 ) ) ;
#25262=CARTESIAN_POINT ( 'NONE',  ( 128.0812361363527998, 241.9574749595457774, 45.00000000000000000 ) ) ;
#25264=PLANE ( 'NONE',  #22152 ) ;
#25266=EDGE_LOOP ( 'NONE', ( #27665, #9739, #7187, #23402 ) ) ;
#25267=CARTESIAN_POINT ( 'NONE',  ( -12.00299901279919723, 223.4254219457707222, 45.00000000000000000 ) ) ;
#25268=ORIENTED_EDGE ( 'NONE', *, *, #19852, .T. ) ;
#25271=ADVANCED_FACE ( 'NONE', ( #24750 ), #20290, .F. ) ;
#25283=CARTESIAN_POINT ( 'NONE',  ( 113.0425250404538673, 226.9187638636466602, 45.00000000000000000 ) ) ;
#25292=VECTOR ( 'NONE', #26070, 1000.000000000000000 ) ;
#25303=ORIENTED_EDGE ( 'NONE', *, *, #21318, .T. ) ;
#25312=VECTOR ( 'NONE', #13408, 1000.000000000000000 ) ;
#25315=AXIS2_PLACEMENT_3D ( 'NONE', #14324, #8419, #14894 ) ;
#25324=ORIENTED_EDGE ( 'NONE', *, *, #13405, .F. ) ;
#25326=LINE ( 'NONE', #13764, #963 ) ;
#25336=FACE_OUTER_BOUND ( 'NONE', #23077, .T. ) ;
#25347=CARTESIAN_POINT ( 'NONE',  ( 25.90578987075423001, -14.95671475544977724, -45.00000000000000000 ) ) ;
#25350=VERTEX_POINT ( 'NONE', #16551 ) ;
#25356=VECTOR ( 'NONE', #5160, 1000.000000000000000 ) ;
#25360=VECTOR ( 'NONE', #27106, 1000.000000000000000 ) ;
#25383=EDGE_CURVE ( 'NONE', #28122, #19128, #1449, .T. ) ;
#25387=ORIENTED_EDGE ( 'NONE', *, *, #26222, .T. ) ;
#25394=LINE ( 'NONE', #8012, #19663 ) ;
#25420=CARTESIAN_POINT ( 'NONE',  ( 115.1711027725237955, 217.3894761555985156, 45.00000000000000000 ) ) ;
#25472=ORIENTED_EDGE ( 'NONE', *, *, #20597, .T. ) ;
#25479=DIRECTION ( 'NONE',  ( -0.000000000000000000, -0.000000000000000000, -1.000000000000000000 ) ) ;
#25498=DIRECTION ( 'NONE',  ( -0.000000000000000000, -0.000000000000000000, -1.000000000000000000 ) ) ;
#25505=DIRECTION ( 'NONE',  ( -0.7440215159219069063, -0.6681556583950086781, 0.000000000000000000 ) ) ;
#25514=EDGE_CURVE ( 'NONE', #27280, #20930, #28007, .T. ) ;
#25518=CARTESIAN_POINT ( 'NONE',  ( 134.9999999999998579, 220.0000000000000284, 45.00000000000000000 ) ) ;
#25536=CARTESIAN_POINT ( 'NONE',  ( 28.57744295357075259, -14.51376905457599342, -45.00000000000000000 ) ) ;
#25538=DIRECTION ( 'NONE',  ( -0.2588190451025321748, -0.9659258262890652036, 0.000000000000000000 ) ) ;
#25543=EDGE_LOOP ( 'NONE', ( #14577, #11220, #18294, #18417 ) ) ;
#25544=CARTESIAN_POINT ( 'NONE',  ( -12.00299901279919723, 223.4254219457707222, 45.00000000000000000 ) ) ;
#25550=ORIENTED_EDGE ( 'NONE', *, *, #17273, .T. ) ;
#25555=ADVANCED_FACE ( 'NONE', ( #21705 ), #23577, .F. ) ;
#25583=CARTESIAN_POINT ( 'NONE',  ( 176.5942101292460222, 101.9567147554491271, -45.00000000000000000 ) ) ;
#25589=CARTESIAN_POINT ( 'NONE',  ( -55.40193461144291831, 169.7519813918499665, 45.00000000000000000 ) ) ;
#25601=ORIENTED_EDGE ( 'NONE', *, *, #18693, .F. ) ;
#25613=AXIS2_PLACEMENT_3D ( 'NONE', #16887, #27791, #19322 ) ;
#25628=EDGE_CURVE ( 'NONE', #5518, #25999, #1868, .T. ) ;
#25650=ORIENTED_EDGE ( 'NONE', *, *, #22501, .T. ) ;
#25668=CARTESIAN_POINT ( 'NONE',  ( 156.9574749595459195, 226.9187638636467739, 45.00000000000000000 ) ) ;
#25680=CARTESIAN_POINT ( 'NONE',  ( 67.86343429515802939, -22.14858123305036486, 45.00000000000000000 ) ) ;
#25710=ORIENTED_EDGE ( 'NONE', *, *, #12060, .T. ) ;
#25715=ORIENTED_EDGE ( 'NONE', *, *, #11615, .T. ) ;
#25719=VECTOR ( 'NONE', #16060, 1000.000000000000000 ) ;
#25721=DIRECTION ( 'NONE',  ( 0.8916010070293515222, 0.4528218681382848443, 0.000000000000000000 ) ) ;
#25749=CARTESIAN_POINT ( 'NONE',  ( 147.3660254037842492, 239.4185842870417673, -45.00000000000000000 ) ) ;
#25761=ORIENTED_EDGE ( 'NONE', *, *, #24894, .T. ) ;
#25774=ORIENTED_EDGE ( 'NONE', *, *, #3674, .T. ) ;
#25781=VERTEX_POINT ( 'NONE', #4104 ) ;
#25784=VECTOR ( 'NONE', #12601, 999.9999999999998863 ) ;
#25801=VECTOR ( 'NONE', #14813, 1000.000000000000114 ) ;
#25814=CARTESIAN_POINT ( 'NONE',  ( 140.5127944162910865, 243.3752990424897575, -45.00000000000000000 ) ) ;
#25832=ORIENTED_EDGE ( 'NONE', *, *, #10850, .T. ) ;
#25859=PRODUCT_CONTEXT ( 'NONE', #4132, 'mechanical' ) ;
#25868=VERTEX_POINT ( 'NONE', #26361 ) ;
#25884=ORIENTED_EDGE ( 'NONE', *, *, #6137, .F. ) ;
#25889=PLANE ( 'NONE',  #13979 ) ;
#25926=CARTESIAN_POINT ( 'NONE',  ( 12.78000883847031588, 237.8887863075477469, 45.00000000000000000 ) ) ;
#25934=ORIENTED_EDGE ( 'NONE', *, *, #22908, .F. ) ;
#25960=DIRECTION ( 'NONE',  ( -0.7071067811865474617, -0.7071067811865474617, 0.000000000000000000 ) ) ;
#25987=DIRECTION ( 'NONE',  ( -0.4528218681383003319, -0.8916010070293436396, 0.000000000000000000 ) ) ;
#25999=VERTEX_POINT ( 'NONE', #2801 ) ;
#26021=EDGE_CURVE ( 'NONE', #9499, #8677, #16321, .T. ) ;
#26023=CARTESIAN_POINT ( 'NONE',  ( 153.4775906502256930, 212.3463313526982859, -45.00000000000000000 ) ) ;
#26034=( LENGTH_UNIT ( ) NAMED_UNIT ( * ) SI_UNIT ( .MILLI., .METRE. ) );
#26038=EDGE_CURVE ( 'NONE', #11330, #5169, #24505, .T. ) ;
#26069=CARTESIAN_POINT ( 'NONE',  ( 145.6339745962154097, 240.4185842870418242, 45.00000000000000000 ) ) ;
#26070=DIRECTION ( 'NONE',  ( -0.2588190451025286221, -0.9659258262890662028, 0.000000000000000000 ) ) ;
#26075=DIRECTION ( 'NONE',  ( 0.6681556583950049033, -0.7440215159219103480, 0.000000000000000000 ) ) ;
#26084=CARTESIAN_POINT ( 'NONE',  ( 115.5814157129579058, 207.6339745962153245, 45.00000000000000000 ) ) ;
#26105=VERTEX_POINT ( 'NONE', #23055 ) ;
#26111=EDGE_CURVE ( 'NONE', #20930, #15999, #23196, .T. ) ;
#26114=EDGE_CURVE ( 'NONE', #24909, #13241, #27488, .T. ) ;
#26124=CARTESIAN_POINT ( 'NONE',  ( 150.8670668058247202, 207.8247714198255949, 45.00000000000000000 ) ) ;
#26129=FACE_OUTER_BOUND ( 'NONE', #6411, .T. ) ;
#26142=EDGE_CURVE ( 'NONE', #11731, #1736, #19023, .T. ) ;
#26154=VECTOR ( 'NONE', #4052, 1000.000000000000114 ) ;
#26199=ADVANCED_FACE ( 'NONE', ( #4208 ), #17708, .F. ) ;
#26222=EDGE_CURVE ( 'NONE', #28003, #21880, #8393, .T. ) ;
#26226=DIRECTION ( 'NONE',  ( -0.9784193629480781862, 0.2066290158914688424, 0.000000000000000000 ) ) ;
#26235=CARTESIAN_POINT ( 'NONE',  ( 127.3463313526980727, 238.4775906502252667, 45.00000000000000000 ) ) ;
#26252=VECTOR ( 'NONE', #19996, 1000.000000000000114 ) ;
#26260=VECTOR ( 'NONE', #25479, 1000.000000000000000 ) ;
#26264=CARTESIAN_POINT ( 'NONE',  ( -10.78991826960876033, 200.8449754580304898, 45.00000000000000000 ) ) ;
#26266=DIRECTION ( 'NONE',  ( 0.8379557447115514313, -0.5457381880580733924, 0.000000000000000000 ) ) ;
#26269=CARTESIAN_POINT ( 'NONE',  ( 157.9999999999998579, 221.0000000000000284, -45.00000000000000000 ) ) ;
#26324=ORIENTED_EDGE ( 'NONE', *, *, #16083, .T. ) ;
#26326=DIRECTION ( 'NONE',  ( 0.5457381880580733924, 0.8379557447115514313, 0.000000000000000000 ) ) ;
#26348=DIRECTION ( 'NONE',  ( 0.2588190451025122463, -0.9659258262890706437, 0.000000000000000000 ) ) ;
#26351=CARTESIAN_POINT ( 'NONE',  ( 48.74042075079900371, -13.05995637893015449, 45.00000000000000000 ) ) ;
#26361=CARTESIAN_POINT ( 'NONE',  ( 114.5814157129578916, 209.3660254037841923, 45.00000000000000000 ) ) ;
#26368=DIRECTION ( 'NONE',  ( 0.2066290158914672603, 0.9784193629480785193, -0.000000000000000000 ) ) ;
#26390=AXIS2_PLACEMENT_3D ( 'NONE', #706, #2412, #7169 ) ;
#26391=VECTOR ( 'NONE', #5756, 1000.000000000000000 ) ;
#26395=ORIENTED_EDGE ( 'NONE', *, *, #9850, .T. ) ;
#26402=UNCERTAINTY_MEASURE_WITH_UNIT (LENGTH_MEASURE( 1.000000000000000082E-05 ), #26034, 'distance_accuracy_value', 'NONE');
#26410=VECTOR ( 'NONE', #8543, 1000.000000000000000 ) ;
#26443=DIRECTION ( 'NONE',  ( 0.3102637045530588500, -0.9506505318133536830, 0.000000000000000000 ) ) ;
#26444=ORIENTED_EDGE ( 'NONE', *, *, #3475, .T. ) ;
#26455=AXIS2_PLACEMENT_3D ( 'NONE', #24466, #2762, #4773 ) ;
#26459=ADVANCED_FACE ( 'NONE', ( #3182 ), #26607, .F. ) ;
#26467=CARTESIAN_POINT ( 'NONE',  ( 130.0130877889309602, 242.4751130497508029, 45.00000000000000000 ) ) ;
#26468=LINE ( 'NONE', #6799, #5430 ) ;
#26479=ORIENTED_EDGE ( 'NONE', *, *, #5266, .F. ) ;
#26480=CARTESIAN_POINT ( 'NONE',  ( 117.5127944162877753, 203.5381304684075019, -45.00000000000000000 ) ) ;
#26481=FACE_OUTER_BOUND ( 'NONE', #6828, .T. ) ;
#26518=VECTOR ( 'NONE', #2558, 1000.000000000000000 ) ;
#26576=CARTESIAN_POINT ( 'NONE',  ( -41.54405845664282282, 46.26118624020713099, 45.00000000000000000 ) ) ;
#26590=DIRECTION ( 'NONE',  ( 0.8379557447115514313, -0.5457381880580733924, 0.000000000000000000 ) ) ;
#26607=PLANE ( 'NONE',  #26455 ) ;
#26652=LINE ( 'NONE', #26235, #14696 ) ;
#26696=DIRECTION ( 'NONE',  ( -0.000000000000000000, -0.000000000000000000, -1.000000000000000000 ) ) ;
#26702=LINE ( 'NONE', #22258, #4632 ) ;
#26710=EDGE_CURVE ( 'NONE', #9201, #194, #26723, .T. ) ;
#26718=ORIENTED_EDGE ( 'NONE', *, *, #24762, .T. ) ;
#26723=LINE ( 'NONE', #4886, #24656 ) ;
#26725=CARTESIAN_POINT ( 'NONE',  ( 137.6105238444007455, 239.8288972274759203, -45.00000000000000000 ) ) ;
#26728=AXIS2_PLACEMENT_3D ( 'NONE', #23385, #16645, #25116 ) ;
#26777=LINE ( 'NONE', #11846, #13784 ) ;
#26790=DIRECTION ( 'NONE',  ( 0.6681556583950252204, 0.7440215159218921404, 0.000000000000000000 ) ) ;
#26795=VERTEX_POINT ( 'NONE', #12503 ) ;
#26796=DIRECTION ( 'NONE',  ( 0.7440215159218921404, -0.6681556583950251094, 0.000000000000000000 ) ) ;
#26799=ORIENTED_EDGE ( 'NONE', *, *, #23039, .T. ) ;
#26811=CARTESIAN_POINT ( 'NONE',  ( 52.57751368840760620, 248.9624084326366358, 45.00000000000000000 ) ) ;
#26814=DIRECTION ( 'NONE',  ( 0.05364526231779759985, 0.9985600561963485777, 0.000000000000000000 ) ) ;
#26834=EDGE_CURVE ( 'NONE', #13479, #14223, #5873, .T. ) ;
#26855=DIRECTION ( 'NONE',  ( -0.2588190451024993122, 0.9659258262890740854, 0.000000000000000000 ) ) ;
#26857=AXIS2_PLACEMENT_3D ( 'NONE', #7505, #1163, #14254 ) ;
#26858=VERTEX_POINT ( 'NONE', #7760 ) ;
#26871=LINE ( 'NONE', #7199, #7401 ) ;
#26889=DIRECTION ( 'NONE',  ( 0.2588190451025121908, -0.9659258262890705327, 0.000000000000000000 ) ) ;
#26891=ORIENTED_EDGE ( 'NONE', *, *, #24433, .T. ) ;
#26893=CARTESIAN_POINT ( 'NONE',  ( 154.8288972274760908, 222.6105238444010297, 45.00000000000000000 ) ) ;
#26899=EDGE_CURVE ( 'NONE', #24769, #24234, #3088, .T. ) ;
#26903=ORIENTED_EDGE ( 'NONE', *, *, #3439, .T. ) ;
#26904=FACE_OUTER_BOUND ( 'NONE', #26905, .T. ) ;
#26905=EDGE_LOOP ( 'NONE', ( #5636, #13746, #11869, #7824, #8525, #10494, #19642, #6992, #13455, #8458, #551, #24304, #9837, #17161, #18189, #14060, #12005, #22646, #4830, #19438, #14720, #22189, #5483, #5439, #25303, #20440, #7369, #24957, #25650, #8244, #15313, #3947, #14065, #22167, #10501, #6786, #26903, #27584, #21944, #9741, #24278, #20984, #10542, #20435, #25268, #2490, #11620, #7613, #23096, #25715, #2870, #1719, #24389, #19025, #10425, #25761, #694, #25550, #8954, #25127, #14925, #3990, #9370, #6495, #1869, #21422, #6740, #24509, #5947, #7721, #16861, #15643 ) ) ;
#26924=VERTEX_POINT ( 'NONE', #4424 ) ;
#26928=EDGE_CURVE ( 'NONE', #13840, #11731, #19377, .T. ) ;
#26942=CARTESIAN_POINT ( 'NONE',  ( 115.1711027725237528, 222.6105238444006886, 45.00000000000000000 ) ) ;
#26959=CARTESIAN_POINT ( 'NONE',  ( 111.9999999999999574, 220.9999999999996874, 45.00000000000000000 ) ) ;
#26970=ORIENTED_EDGE ( 'NONE', *, *, #16374, .F. ) ;
#26973=EDGE_LOOP ( 'NONE', ( #7709, #21973, #8318, #14224 ) ) ;
#26984=VECTOR ( 'NONE', #22327, 1000.000000000000000 ) ;
#27003=VECTOR ( 'NONE', #16611, 1000.000000000000000 ) ;
#27004=PLANE ( 'NONE',  #18476 ) ;
#27006=VECTOR ( 'NONE', #11270, 1000.000000000000000 ) ;
#27012=LINE ( 'NONE', #9214, #11926 ) ;
#27013=DIRECTION ( 'NONE',  ( -0.8916010070293547418, -0.4528218681382785715, 0.000000000000000000 ) ) ;
#27019=EDGE_CURVE ( 'NONE', #3365, #20790, #19799, .T. ) ;
#27065=CARTESIAN_POINT ( 'NONE',  ( 74.37710191228967460, 227.8920494084358950, -45.00000000000000000 ) ) ;
#27068=ORIENTED_EDGE ( 'NONE', *, *, #2890, .T. ) ;
#27072=EDGE_CURVE ( 'NONE', #16719, #999, #1274, .T. ) ;
#27092=CARTESIAN_POINT ( 'NONE',  ( 141.9187638636469160, 241.9574749595457774, 45.00000000000000000 ) ) ;
#27096=FACE_OUTER_BOUND ( 'NONE', #22668, .T. ) ;
#27098=VECTOR ( 'NONE', #21464, 1000.000000000000000 ) ;
#27106=DIRECTION ( 'NONE',  ( -0.2066290158914688424, -0.9784193629480781862, 0.000000000000000000 ) ) ;
#27121=EDGE_CURVE ( 'NONE', #502, #19228, #4705, .T. ) ;
#27141=VECTOR ( 'NONE', #21910, 1000.000000000000114 ) ;
#27189=PLANE ( 'NONE',  #11230 ) ;
#27205=CARTESIAN_POINT ( 'NONE',  ( 146.9844428835009467, 225.6878133005969858, -45.00000000000000000 ) ) ;
#27234=ORIENTED_EDGE ( 'NONE', *, *, #9623, .T. ) ;
#27240=ORIENTED_EDGE ( 'NONE', *, *, #23253, .T. ) ;
#27241=EDGE_CURVE ( 'NONE', #22164, #18948, #14482, .T. ) ;
#27262=LINE ( 'NONE', #7599, #19999 ) ;
#27271=EDGE_LOOP ( 'NONE', ( #19316, #12488, #11450, #6479 ) ) ;
#27280=VERTEX_POINT ( 'NONE', #5285 ) ;
#27281=EDGE_CURVE ( 'NONE', #6349, #13016, #22816, .T. ) ;
#27310=VECTOR ( 'NONE', #23910, 1000.000000000000000 ) ;
#27332=CARTESIAN_POINT ( 'NONE',  ( 116.5224093497742786, 212.3463313526978595, 45.00000000000000000 ) ) ;
#27342=VERTEX_POINT ( 'NONE', #5709 ) ;
#27354=VECTOR ( 'NONE', #26814, 999.9999999999998863 ) ;
#27361=DIRECTION ( 'NONE',  ( -0.000000000000000000, -0.000000000000000000, -1.000000000000000000 ) ) ;
#27372=FACE_OUTER_BOUND ( 'NONE', #25028, .T. ) ;
#27400=LINE ( 'NONE', #25262, #2721 ) ;
#27407=FACE_OUTER_BOUND ( 'NONE', #7725, .T. ) ;
#27421=EDGE_CURVE ( 'NONE', #13840, #8625, #23660, .T. ) ;
#27423=EDGE_CURVE ( 'NONE', #4484, #11107, #5986, .T. ) ;
#27431=CARTESIAN_POINT ( 'NONE',  ( 154.4185842870420799, 207.6339745962155803, 45.00000000000000000 ) ) ;
#27456=CARTESIAN_POINT ( 'NONE',  ( 140.5127944162910865, 243.3752990424897575, 45.00000000000000000 ) ) ;
#27460=EDGE_CURVE ( 'NONE', #10156, #23257, #12615, .T. ) ;
#27469=LINE ( 'NONE', #11716, #11191 ) ;
#27470=VERTEX_POINT ( 'NONE', #25040 ) ;
#27475=CARTESIAN_POINT ( 'NONE',  ( 69.99612328191057031, 261.2290884209365345, 45.00000000000000000 ) ) ;
#27488=LINE ( 'NONE', #12155, #23708 ) ;
#27511=CARTESIAN_POINT ( 'NONE',  ( 146.9844428835009467, 225.6878133005969858, 45.00000000000000000 ) ) ;
#27518=CARTESIAN_POINT ( 'NONE',  ( 95.82124051657368113, -20.23615780638419182, 45.00000000000000000 ) ) ;
#27521=ORIENTED_EDGE ( 'NONE', *, *, #10141, .F. ) ;
#27545=DIRECTION ( 'NONE',  ( -0.000000000000000000, -0.000000000000000000, -1.000000000000000000 ) ) ;
#27584=ORIENTED_EDGE ( 'NONE', *, *, #20197, .T. ) ;
#27586=ADVANCED_FACE ( 'NONE', ( #25170 ), #16559, .F. ) ;
#27612=LINE ( 'NONE', #16855, #1782 ) ;
#27618=ORIENTED_EDGE ( 'NONE', *, *, #24053, .F. ) ;
#27628=EDGE_CURVE ( 'NONE', #13016, #8625, #23161, .T. ) ;
#27645=LINE ( 'NONE', #19039, #27003 ) ;
#27665=ORIENTED_EDGE ( 'NONE', *, *, #20647, .T. ) ;
#27680=LINE ( 'NONE', #25536, #7864 ) ;
#27689=LINE ( 'NONE', #25544, #7905 ) ;
#27691=VERTEX_POINT ( 'NONE', #13531 ) ;
#27696=EDGE_CURVE ( 'NONE', #25999, #7120, #27012, .T. ) ;
#27697=VERTEX_POINT ( 'NONE', #9505 ) ;
#27708=AXIS2_PLACEMENT_3D ( 'NONE', #25589, #21144, #7936 ) ;
#27725=EDGE_CURVE ( 'NONE', #27697, #7120, #7346, .T. ) ;
#27729=EDGE_LOOP ( 'NONE', ( #10293, #19541, #9847, #18063 ) ) ;
#27731=ADVANCED_FACE ( 'NONE', ( #18262 ), #22282, .F. ) ;
#27740=LINE ( 'NONE', #13079, #21365 ) ;
#27755=EDGE_CURVE ( 'NONE', #5560, #15143, #13677, .T. ) ;
#27761=CARTESIAN_POINT ( 'NONE',  ( 119.1329331941752230, 232.1752285801739220, 45.00000000000000000 ) ) ;
#27762=AXIS2_PLACEMENT_3D ( 'NONE', #15577, #21890, #13282 ) ;
#27763=ORIENTED_EDGE ( 'NONE', *, *, #3460, .F. ) ;
#27791=DIRECTION ( 'NONE',  ( -0.8379557447115515423, 0.5457381880580733924, 0.000000000000000000 ) ) ;
#27800=DIRECTION ( 'NONE',  ( 0.9659258262890662028, -0.2588190451025286221, 0.000000000000000000 ) ) ;
#27803=ORIENTED_EDGE ( 'NONE', *, *, #15149, .F. ) ;
#27813=LINE ( 'NONE', #20658, #11413 ) ;
#27820=CARTESIAN_POINT ( 'NONE',  ( 128.0812361363527998, 241.9574749595457774, 45.00000000000000000 ) ) ;
#27838=DIRECTION ( 'NONE',  ( 1.000000000000000000, 0.000000000000000000, 0.000000000000000000 ) ) ;
#27846=DIRECTION ( 'NONE',  ( 1.000000000000000000, 0.000000000000000000, 0.000000000000000000 ) ) ;
#27849=DIRECTION ( 'NONE',  ( 0.9784193629480785193, -0.2066290158914672881, 0.000000000000000000 ) ) ;
#27861=AXIS2_PLACEMENT_3D ( 'NONE', #4575, #10772, #21538 ) ;
#27870=DIRECTION ( 'NONE',  ( 0.4999999999999985012, -0.8660254037844394848, 0.000000000000000000 ) ) ;
#27872=CARTESIAN_POINT ( 'NONE',  ( 147.1752285801741493, 235.8670668058244644, 45.00000000000000000 ) ) ;
#27895=ORIENTED_EDGE ( 'NONE', *, *, #26928, .F. ) ;
#27917=ORIENTED_EDGE ( 'NONE', *, *, #109, .F. ) ;
#27920=CARTESIAN_POINT ( 'NONE',  ( 136.0000000000000853, 196.9999999999997442, 45.00000000000000000 ) ) ;
#27934=DIRECTION ( 'NONE',  ( -0.8660254037844394848, -0.4999999999999985012, 0.000000000000000000 ) ) ;
#27935=ORIENTED_EDGE ( 'NONE', *, *, #13063, .F. ) ;
#27936=FACE_OUTER_BOUND ( 'NONE', #28261, .T. ) ;
#27939=ORIENTED_EDGE ( 'NONE', *, *, #26142, .F. ) ;
#27942=AXIS2_PLACEMENT_3D ( 'NONE', #16978, #1183, #23586 ) ;
#27988=LINE ( 'NONE', #8327, #14258 ) ;
#27997=VERTEX_POINT ( 'NONE', #7846 ) ;
#28003=VERTEX_POINT ( 'NONE', #8275 ) ;
#28007=LINE ( 'NONE', #12677, #4880 ) ;
#28016=VERTEX_POINT ( 'NONE', #4095 ) ;
#28022=PLANE ( 'NONE',  #17934 ) ;
#28024=ORIENTED_EDGE ( 'NONE', *, *, #15800, .F. ) ;
#28028=DIRECTION ( 'NONE',  ( 0.7071067811865335839, -0.7071067811865613395, 0.000000000000000000 ) ) ;
#28063=PLANE ( 'NONE',  #12921 ) ;
#28071=DIRECTION ( 'NONE',  ( 0.8660254037844394848, 0.4999999999999985012, 0.000000000000000000 ) ) ;
#28087=ORIENTED_EDGE ( 'NONE', *, *, #109, .T. ) ;
#28111=AXIS2_PLACEMENT_3D ( 'NONE', #18062, #9009, #16058 ) ;
#28122=VERTEX_POINT ( 'NONE', #24072 ) ;
#28127=EDGE_CURVE ( 'NONE', #6015, #10156, #17176, .T. ) ;
#28132=LINE ( 'NONE', #16949, #6646 ) ;
#28147=EDGE_CURVE ( 'NONE', #23933, #9172, #17310, .T. ) ;
#28154=EDGE_LOOP ( 'NONE', ( #20894, #18222, #1631, #612 ) ) ;
#28166=VECTOR ( 'NONE', #13769, 999.9999999999998863 ) ;
#28186=VERTEX_POINT ( 'NONE', #5090 ) ;
#28210=EDGE_LOOP ( 'NONE', ( #21097, #10782, #19376, #1596 ) ) ;
#28230=EDGE_LOOP ( 'NONE', ( #24877, #10762, #15759, #22088 ) ) ;
#28238=ADVANCED_FACE ( 'NONE', ( #15893 ), #24493, .F. ) ;
#28261=EDGE_LOOP ( 'NONE', ( #4313, #15502, #9668, #15818 ) ) ;
#28273=CARTESIAN_POINT ( 'NONE',  ( 124.9999999999998579, 220.0000000000000284, 45.00000000000000000 ) ) ;
#28284=EDGE_CURVE ( 'NONE', #15009, #4982, #7403, .T. ) ;
#28328=ORIENTED_EDGE ( 'NONE', *, *, #13321, .F. ) ;
#28336=LINE ( 'NONE', #6517, #8439 ) ;
#28340=ORIENTED_EDGE ( 'NONE', *, *, #23253, .F. ) ;
#28362=ORIENTED_EDGE ( 'NONE', *, *, #24762, .F. ) ;
#28368=CARTESIAN_POINT ( 'NONE',  ( 47.90501010967909679, 226.8374036014029969, 45.00000000000000000 ) ) ;
#28380=ORIENTED_EDGE ( 'NONE', *, *, #21386, .F. ) ;
#28421=COLOUR_RGB('Light Blue',0.38,0.62,0.78);
#28422=FILL_AREA_STYLE_COLOUR('',#28421);
#28423=FILL_AREA_STYLE('',(#28422));
#28424=SURFACE_STYLE_FILL_AREA(#28423);
#28425=SURFACE_SIDE_STYLE('',(#28424));
#28426=SURFACE_STYLE_USAGE(.BOTH.,#28425);
#28427=PRESENTATION_STYLE_ASSIGNMENT((#28426));
ENDSEC;
END-ISO-10303-21;
